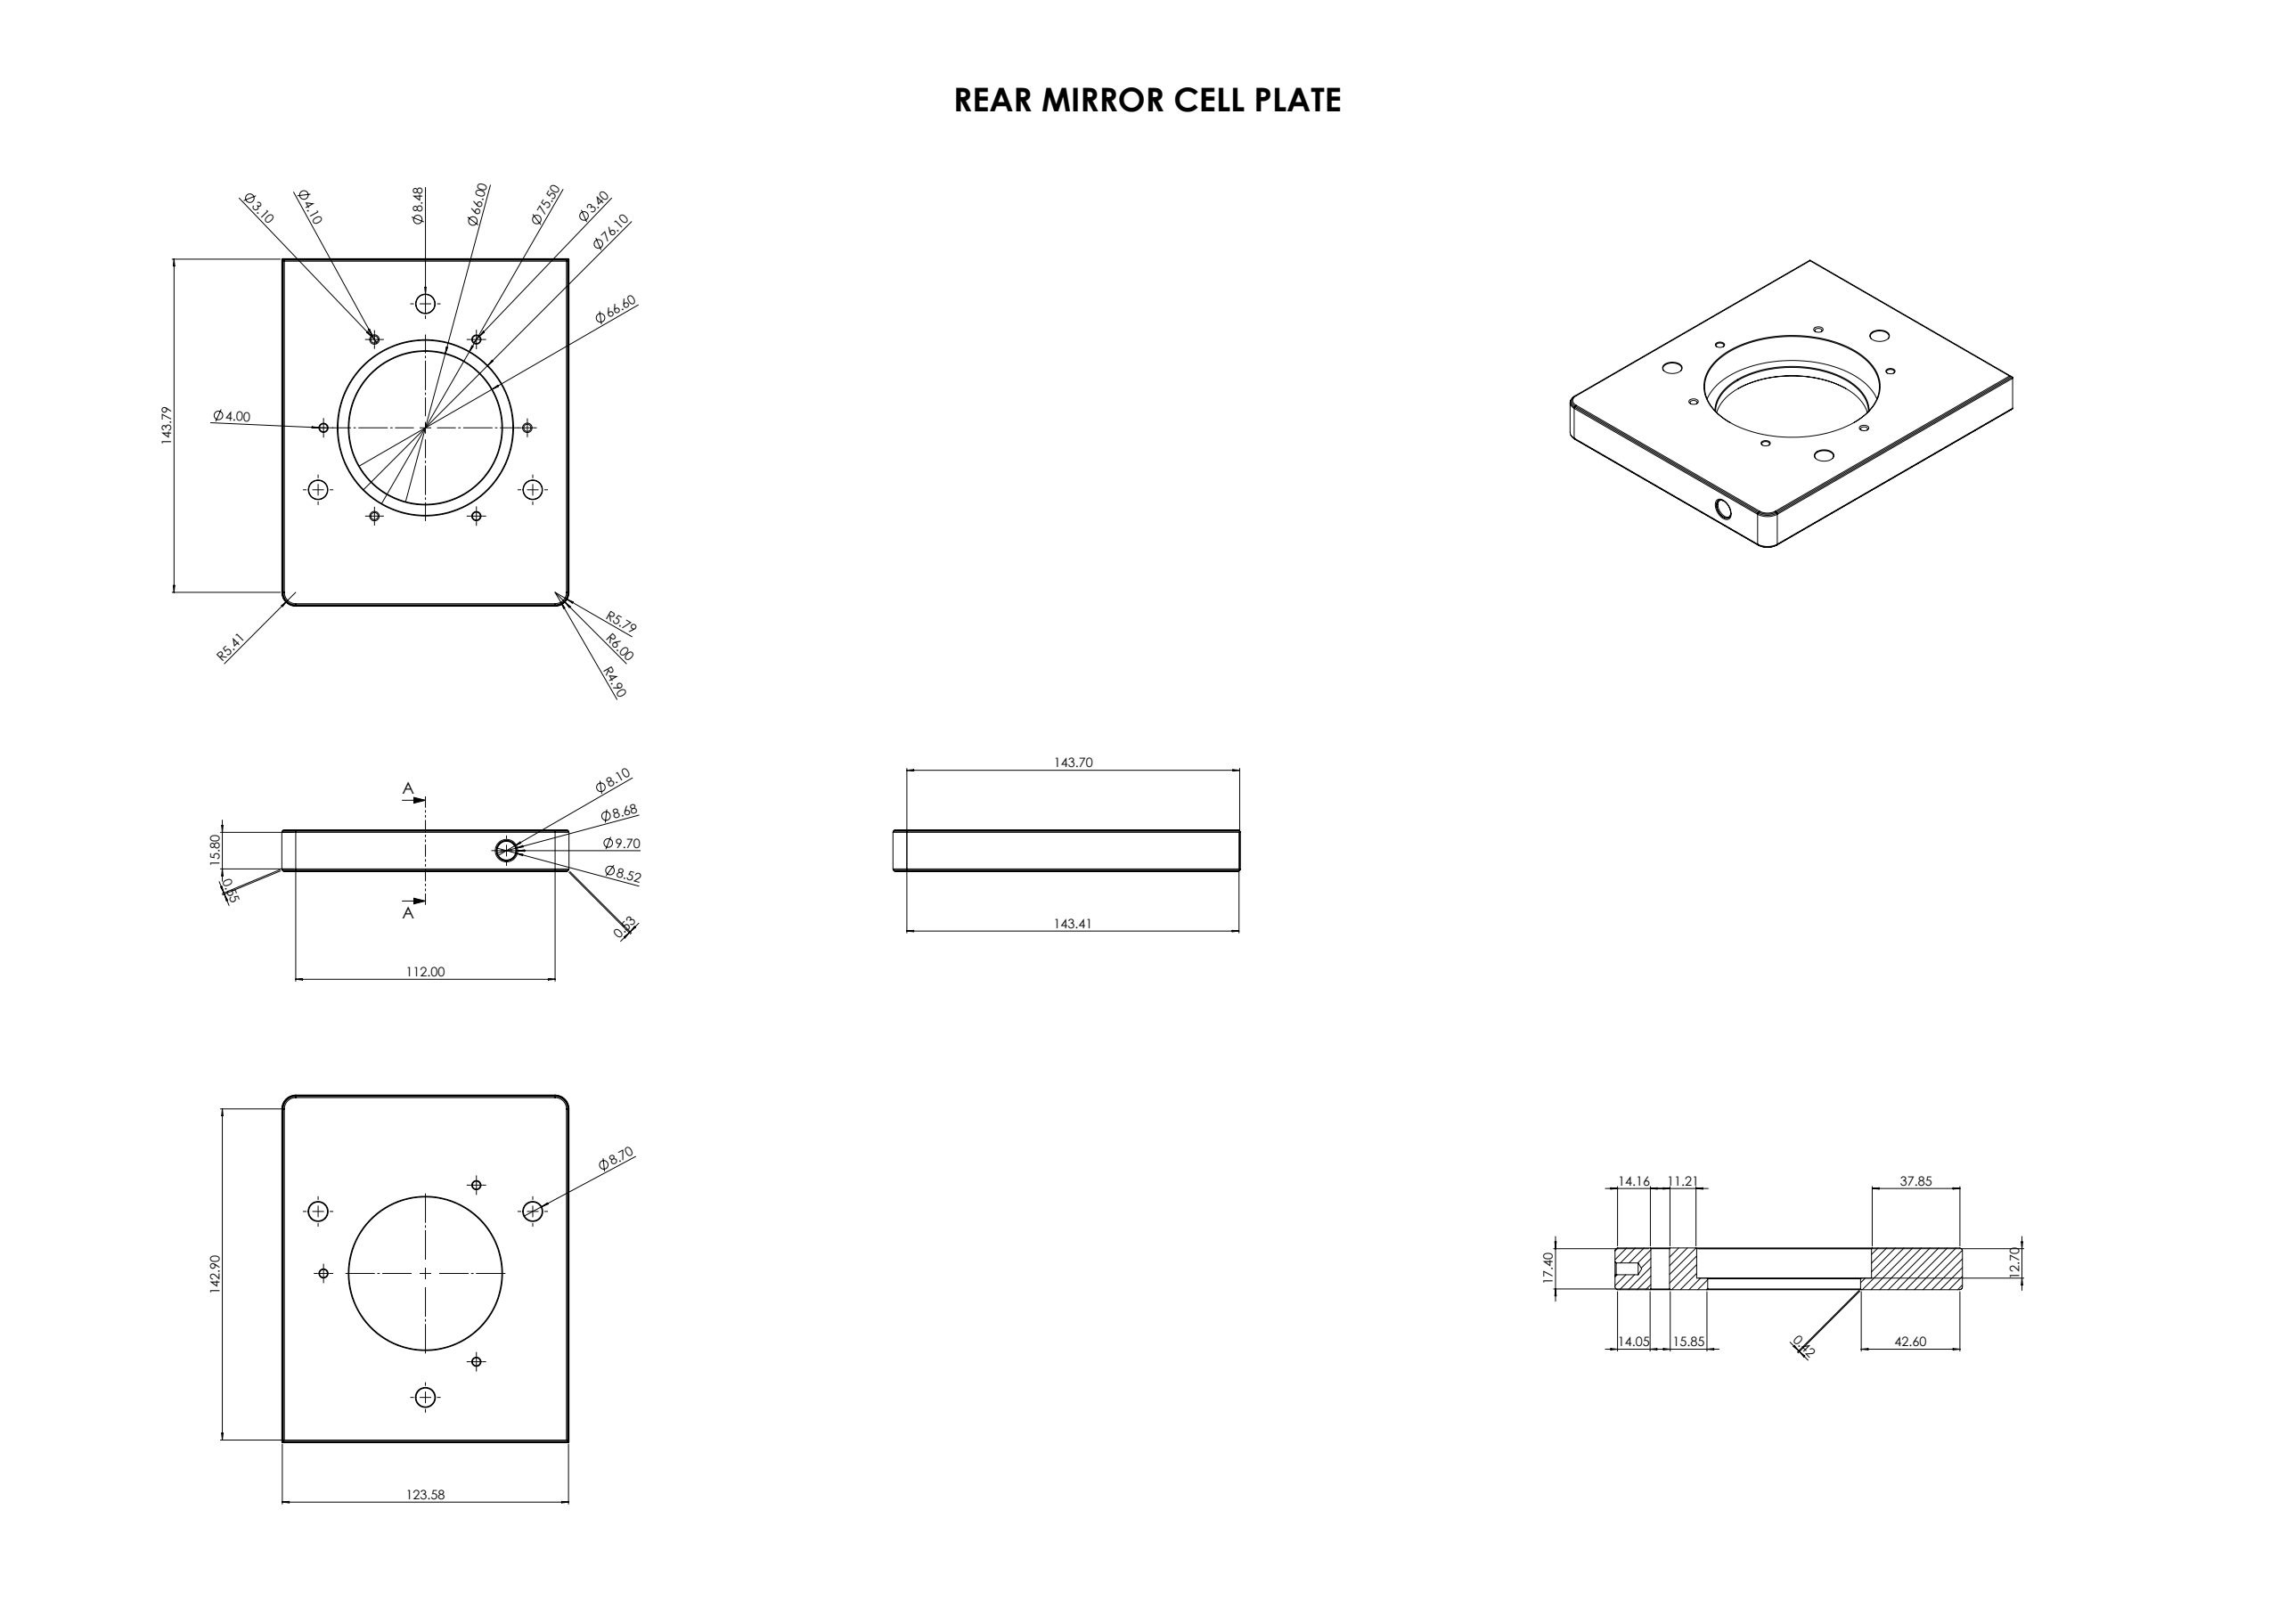
ISO-10303-21;
HEADER;
/* Generated by software containing ST-Developer
 * from STEP Tools, Inc. (www.steptools.com) 
 */

FILE_DESCRIPTION(
/* description */ (''),
/* implementation_level */ '2;1');

FILE_NAME(
/* name */ '02_Rear_Mirror_Cell_Plate.step',
/* time_stamp */ '2026-10-19T22:59:19-07:00',
/* author */ (''),
/* organization */ (''),
/* preprocessor_version */ 'ST-DEVELOPER v20.2',
/* originating_system */ 'Autodesk Translation Framework v15.15.0.0',
/* authorisation */ '');

FILE_SCHEMA (('AUTOMOTIVE_DESIGN { 1 0 10303 214 3 1 1 }'));
ENDSEC;

DATA;
#10=MECHANICAL_DESIGN_GEOMETRIC_PRESENTATION_REPRESENTATION('',(#912),#53650);
#880=SHAPE_REPRESENTATION_RELATIONSHIP('SRR','None',#53725,#896);
#896=ADVANCED_BREP_SHAPE_REPRESENTATION('',(#928),#53635);
#912=STYLED_ITEM('',(#53944),#928);
#928=MANIFOLD_SOLID_BREP('Rear Mirror Cell Plate',#23304);
#961=CYLINDRICAL_SURFACE('',#23742,0.6);
#962=CYLINDRICAL_SURFACE('',#23768,3.3);
#963=CYLINDRICAL_SURFACE('',#23773,3.775);
#964=CYLINDRICAL_SURFACE('',#23781,0.17);
#965=CYLINDRICAL_SURFACE('',#23787,0.17);
#966=CYLINDRICAL_SURFACE('',#23793,0.17);
#967=CYLINDRICAL_SURFACE('',#23798,0.405);
#968=CYLINDRICAL_SURFACE('',#23802,0.404999999999999);
#969=CYLINDRICAL_SURFACE('',#23806,0.405);
#970=CYLINDRICAL_SURFACE('',#23818,0.405);
#971=CYLINDRICAL_SURFACE('',#23823,0.255);
#972=CYLINDRICAL_SURFACE('',#23828,0.255);
#973=CYLINDRICAL_SURFACE('',#23833,0.255);
#974=CYLINDRICAL_SURFACE('',#23841,0.155);
#975=CYLINDRICAL_SURFACE('',#23846,0.155);
#976=CYLINDRICAL_SURFACE('',#23851,0.155);
#977=CYLINDRICAL_SURFACE('',#23855,0.6);
#1298=FACE_BOUND('',#3695,.T.);
#1299=FACE_BOUND('',#3696,.T.);
#1300=FACE_BOUND('',#3697,.T.);
#1301=FACE_BOUND('',#3698,.T.);
#1302=FACE_BOUND('',#3699,.T.);
#1303=FACE_BOUND('',#3700,.T.);
#1304=FACE_BOUND('',#3701,.T.);
#1305=FACE_BOUND('',#3704,.T.);
#1306=FACE_BOUND('',#3705,.T.);
#1307=FACE_BOUND('',#3706,.T.);
#1308=FACE_BOUND('',#3738,.T.);
#1309=FACE_BOUND('',#3739,.T.);
#1310=FACE_BOUND('',#3740,.T.);
#1311=FACE_BOUND('',#3741,.T.);
#1312=FACE_BOUND('',#3742,.T.);
#1313=FACE_BOUND('',#3743,.T.);
#1314=FACE_BOUND('',#3744,.T.);
#1315=FACE_BOUND('',#3745,.T.);
#1316=FACE_BOUND('',#3746,.T.);
#1317=FACE_BOUND('',#3747,.T.);
#1318=FACE_BOUND('',#3754,.T.);
#1319=FACE_BOUND('',#3773,.T.);
#1485=PLANE('',#23687);
#1486=PLANE('',#23688);
#1487=PLANE('',#23692);
#1488=PLANE('',#23696);
#1489=PLANE('',#23699);
#1490=PLANE('',#23700);
#1491=PLANE('',#23701);
#1492=PLANE('',#23709);
#1493=PLANE('',#23710);
#1494=PLANE('',#23714);
#1495=PLANE('',#23715);
#1496=PLANE('',#23716);
#1497=PLANE('',#23719);
#1498=PLANE('',#23723);
#1499=PLANE('',#23725);
#1500=PLANE('',#23726);
#1501=PLANE('',#23727);
#1502=PLANE('',#23728);
#1503=PLANE('',#23729);
#1504=PLANE('',#23730);
#1505=PLANE('',#23734);
#1506=PLANE('',#23740);
#1507=PLANE('',#23741);
#1508=PLANE('',#23743);
#1509=PLANE('',#23744);
#1510=PLANE('',#23745);
#1511=PLANE('',#23748);
#1512=PLANE('',#23752);
#1513=PLANE('',#23754);
#1514=PLANE('',#23755);
#1515=PLANE('',#23777);
#1516=PLANE('',#23814);
#1517=PLANE('',#23854);
#2336=FACE_OUTER_BOUND('',#3685,.T.);
#2337=FACE_OUTER_BOUND('',#3686,.T.);
#2338=FACE_OUTER_BOUND('',#3687,.T.);
#2339=FACE_OUTER_BOUND('',#3688,.T.);
#2340=FACE_OUTER_BOUND('',#3689,.T.);
#2341=FACE_OUTER_BOUND('',#3690,.T.);
#2342=FACE_OUTER_BOUND('',#3691,.T.);
#2343=FACE_OUTER_BOUND('',#3692,.T.);
#2344=FACE_OUTER_BOUND('',#3693,.T.);
#2345=FACE_OUTER_BOUND('',#3694,.T.);
#2346=FACE_OUTER_BOUND('',#3702,.T.);
#2347=FACE_OUTER_BOUND('',#3703,.T.);
#2348=FACE_OUTER_BOUND('',#3707,.T.);
#2349=FACE_OUTER_BOUND('',#3708,.T.);
#2350=FACE_OUTER_BOUND('',#3709,.T.);
#2351=FACE_OUTER_BOUND('',#3710,.T.);
#2352=FACE_OUTER_BOUND('',#3711,.T.);
#2353=FACE_OUTER_BOUND('',#3712,.T.);
#2354=FACE_OUTER_BOUND('',#3713,.T.);
#2355=FACE_OUTER_BOUND('',#3714,.T.);
#2356=FACE_OUTER_BOUND('',#3715,.T.);
#2357=FACE_OUTER_BOUND('',#3716,.T.);
#2358=FACE_OUTER_BOUND('',#3717,.T.);
#2359=FACE_OUTER_BOUND('',#3718,.T.);
#2360=FACE_OUTER_BOUND('',#3719,.T.);
#2361=FACE_OUTER_BOUND('',#3720,.T.);
#2362=FACE_OUTER_BOUND('',#3721,.T.);
#2363=FACE_OUTER_BOUND('',#3722,.T.);
#2364=FACE_OUTER_BOUND('',#3723,.T.);
#2365=FACE_OUTER_BOUND('',#3724,.T.);
#2366=FACE_OUTER_BOUND('',#3725,.T.);
#2367=FACE_OUTER_BOUND('',#3726,.T.);
#2368=FACE_OUTER_BOUND('',#3727,.T.);
#2369=FACE_OUTER_BOUND('',#3728,.T.);
#2370=FACE_OUTER_BOUND('',#3729,.T.);
#2371=FACE_OUTER_BOUND('',#3730,.T.);
#2372=FACE_OUTER_BOUND('',#3731,.T.);
#2373=FACE_OUTER_BOUND('',#3732,.T.);
#2374=FACE_OUTER_BOUND('',#3733,.T.);
#2375=FACE_OUTER_BOUND('',#3734,.T.);
#2376=FACE_OUTER_BOUND('',#3735,.T.);
#2377=FACE_OUTER_BOUND('',#3736,.T.);
#2378=FACE_OUTER_BOUND('',#3737,.T.);
#2379=FACE_OUTER_BOUND('',#3748,.T.);
#2380=FACE_OUTER_BOUND('',#3749,.T.);
#2381=FACE_OUTER_BOUND('',#3750,.T.);
#2382=FACE_OUTER_BOUND('',#3751,.T.);
#2383=FACE_OUTER_BOUND('',#3752,.T.);
#2384=FACE_OUTER_BOUND('',#3753,.T.);
#2385=FACE_OUTER_BOUND('',#3755,.T.);
#2386=FACE_OUTER_BOUND('',#3756,.T.);
#2387=FACE_OUTER_BOUND('',#3757,.T.);
#2388=FACE_OUTER_BOUND('',#3758,.T.);
#2389=FACE_OUTER_BOUND('',#3759,.T.);
#2390=FACE_OUTER_BOUND('',#3760,.T.);
#2391=FACE_OUTER_BOUND('',#3761,.T.);
#2392=FACE_OUTER_BOUND('',#3762,.T.);
#2393=FACE_OUTER_BOUND('',#3763,.T.);
#2394=FACE_OUTER_BOUND('',#3764,.T.);
#2395=FACE_OUTER_BOUND('',#3765,.T.);
#2396=FACE_OUTER_BOUND('',#3766,.T.);
#2397=FACE_OUTER_BOUND('',#3767,.T.);
#2398=FACE_OUTER_BOUND('',#3768,.T.);
#2399=FACE_OUTER_BOUND('',#3769,.T.);
#2400=FACE_OUTER_BOUND('',#3770,.T.);
#2401=FACE_OUTER_BOUND('',#3771,.T.);
#2402=FACE_OUTER_BOUND('',#3772,.T.);
#2403=FACE_OUTER_BOUND('',#3774,.T.);
#2404=FACE_OUTER_BOUND('',#3775,.T.);
#2405=FACE_OUTER_BOUND('',#3776,.T.);
#2406=FACE_OUTER_BOUND('',#3777,.T.);
#2407=FACE_OUTER_BOUND('',#3778,.T.);
#2408=FACE_OUTER_BOUND('',#3779,.T.);
#2409=FACE_OUTER_BOUND('',#3780,.T.);
#2410=FACE_OUTER_BOUND('',#3781,.T.);
#2411=FACE_OUTER_BOUND('',#3782,.T.);
#2412=FACE_OUTER_BOUND('',#3783,.T.);
#2413=FACE_OUTER_BOUND('',#3784,.T.);
#2414=FACE_OUTER_BOUND('',#3785,.T.);
#2415=FACE_OUTER_BOUND('',#3786,.T.);
#2416=FACE_OUTER_BOUND('',#3787,.T.);
#2417=FACE_OUTER_BOUND('',#3788,.T.);
#2418=FACE_OUTER_BOUND('',#3789,.T.);
#2419=FACE_OUTER_BOUND('',#3790,.T.);
#2420=FACE_OUTER_BOUND('',#3791,.T.);
#2421=FACE_OUTER_BOUND('',#3792,.T.);
#2422=FACE_OUTER_BOUND('',#3793,.T.);
#2423=FACE_OUTER_BOUND('',#3794,.T.);
#2424=FACE_OUTER_BOUND('',#3795,.T.);
#2425=FACE_OUTER_BOUND('',#3796,.T.);
#2426=FACE_OUTER_BOUND('',#3797,.T.);
#2427=FACE_OUTER_BOUND('',#3798,.T.);
#2428=FACE_OUTER_BOUND('',#3799,.T.);
#3685=EDGE_LOOP('',(#15489,#15490,#15491,#15492));
#3686=EDGE_LOOP('',(#15493,#15494,#15495,#15496));
#3687=EDGE_LOOP('',(#15497,#15498,#15499,#15500));
#3688=EDGE_LOOP('',(#15501,#15502,#15503,#15504));
#3689=EDGE_LOOP('',(#15505,#15506,#15507,#15508));
#3690=EDGE_LOOP('',(#15509,#15510,#15511,#15512));
#3691=EDGE_LOOP('',(#15513,#15514,#15515,#15516));
#3692=EDGE_LOOP('',(#15517,#15518,#15519,#15520));
#3693=EDGE_LOOP('',(#15521,#15522,#15523,#15524));
#3694=EDGE_LOOP('',(#15525,#15526,#15527,#15528,#15529,#15530));
#3695=EDGE_LOOP('',(#15531));
#3696=EDGE_LOOP('',(#15532));
#3697=EDGE_LOOP('',(#15533));
#3698=EDGE_LOOP('',(#15534));
#3699=EDGE_LOOP('',(#15535));
#3700=EDGE_LOOP('',(#15536));
#3701=EDGE_LOOP('',(#15537));
#3702=EDGE_LOOP('',(#15538,#15539,#15540,#15541,#15542,#15543));
#3703=EDGE_LOOP('',(#15544,#15545,#15546,#15547));
#3704=EDGE_LOOP('',(#15548));
#3705=EDGE_LOOP('',(#15549));
#3706=EDGE_LOOP('',(#15550));
#3707=EDGE_LOOP('',(#15551,#15552,#15553,#15554,#15555,#15556));
#3708=EDGE_LOOP('',(#15557,#15558,#15559,#15560,#15561));
#3709=EDGE_LOOP('',(#15562,#15563,#15564,#15565,#15566));
#3710=EDGE_LOOP('',(#15567,#15568,#15569,#15570));
#3711=EDGE_LOOP('',(#15571,#15572,#15573,#15574));
#3712=EDGE_LOOP('',(#15575,#15576,#15577,#15578));
#3713=EDGE_LOOP('',(#15579,#15580,#15581,#15582));
#3714=EDGE_LOOP('',(#15583,#15584,#15585,#15586));
#3715=EDGE_LOOP('',(#15587,#15588,#15589,#15590));
#3716=EDGE_LOOP('',(#15591,#15592,#15593,#15594,#15595,#15596));
#3717=EDGE_LOOP('',(#15597,#15598,#15599,#15600,#15601,#15602));
#3718=EDGE_LOOP('',(#15603,#15604,#15605,#15606));
#3719=EDGE_LOOP('',(#15607,#15608,#15609,#15610,#15611));
#3720=EDGE_LOOP('',(#15612,#15613,#15614,#15615,#15616));
#3721=EDGE_LOOP('',(#15617,#15618,#15619,#15620));
#3722=EDGE_LOOP('',(#15621,#15622,#15623,#15624));
#3723=EDGE_LOOP('',(#15625,#15626,#15627,#15628));
#3724=EDGE_LOOP('',(#15629,#15630,#15631,#15632));
#3725=EDGE_LOOP('',(#15633,#15634,#15635,#15636));
#3726=EDGE_LOOP('',(#15637,#15638,#15639,#15640));
#3727=EDGE_LOOP('',(#15641,#15642,#15643,#15644));
#3728=EDGE_LOOP('',(#15645,#15646,#15647,#15648));
#3729=EDGE_LOOP('',(#15649,#15650,#15651,#15652));
#3730=EDGE_LOOP('',(#15653,#15654,#15655,#15656));
#3731=EDGE_LOOP('',(#15657,#15658,#15659,#15660));
#3732=EDGE_LOOP('',(#15661,#15662,#15663,#15664));
#3733=EDGE_LOOP('',(#15665,#15666,#15667,#15668));
#3734=EDGE_LOOP('',(#15669,#15670,#15671,#15672));
#3735=EDGE_LOOP('',(#15673,#15674,#15675,#15676));
#3736=EDGE_LOOP('',(#15677,#15678,#15679,#15680));
#3737=EDGE_LOOP('',(#15681,#15682,#15683,#15684,#15685,#15686));
#3738=EDGE_LOOP('',(#15687));
#3739=EDGE_LOOP('',(#15688));
#3740=EDGE_LOOP('',(#15689));
#3741=EDGE_LOOP('',(#15690));
#3742=EDGE_LOOP('',(#15691));
#3743=EDGE_LOOP('',(#15692));
#3744=EDGE_LOOP('',(#15693));
#3745=EDGE_LOOP('',(#15694));
#3746=EDGE_LOOP('',(#15695));
#3747=EDGE_LOOP('',(#15696));
#3748=EDGE_LOOP('',(#15697,#15698,#15699,#15700));
#3749=EDGE_LOOP('',(#15701,#15702,#15703,#15704));
#3750=EDGE_LOOP('',(#15705,#15706,#15707,#15708,#15709));
#3751=EDGE_LOOP('',(#15710,#15711,#15712,#15713,#15714));
#3752=EDGE_LOOP('',(#15715,#15716,#15717,#15718));
#3753=EDGE_LOOP('',(#15719));
#3754=EDGE_LOOP('',(#15720));
#3755=EDGE_LOOP('',(#15721,#15722,#15723,#15724,#15725));
#3756=EDGE_LOOP('',(#15726,#15727,#15728,#15729,#15730));
#3757=EDGE_LOOP('',(#15731,#15732,#15733,#15734));
#3758=EDGE_LOOP('',(#15735,#15736,#15737,#15738,#15739));
#3759=EDGE_LOOP('',(#15740,#15741,#15742,#15743,#15744));
#3760=EDGE_LOOP('',(#15745,#15746,#15747,#15748));
#3761=EDGE_LOOP('',(#15749,#15750,#15751,#15752,#15753));
#3762=EDGE_LOOP('',(#15754,#15755,#15756,#15757,#15758));
#3763=EDGE_LOOP('',(#15759,#15760,#15761,#15762));
#3764=EDGE_LOOP('',(#15763,#15764,#15765,#15766));
#3765=EDGE_LOOP('',(#15767,#15768,#15769,#15770));
#3766=EDGE_LOOP('',(#15771,#15772,#15773,#15774));
#3767=EDGE_LOOP('',(#15775,#15776,#15777,#15778));
#3768=EDGE_LOOP('',(#15779,#15780,#15781,#15782));
#3769=EDGE_LOOP('',(#15783,#15784,#15785,#15786));
#3770=EDGE_LOOP('',(#15787,#15788,#15789,#15790));
#3771=EDGE_LOOP('',(#15791,#15792,#15793,#15794,#15795));
#3772=EDGE_LOOP('',(#15796,#15797,#15798,#15799));
#3773=EDGE_LOOP('',(#15800));
#3774=EDGE_LOOP('',(#15801,#15802,#15803,#15804,#15805,#15806));
#3775=EDGE_LOOP('',(#15807,#15808,#15809,#15810,#15811));
#3776=EDGE_LOOP('',(#15812,#15813,#15814));
#3777=EDGE_LOOP('',(#15815,#15816,#15817));
#3778=EDGE_LOOP('',(#15818,#15819,#15820,#15821));
#3779=EDGE_LOOP('',(#15822,#15823,#15824,#15825));
#3780=EDGE_LOOP('',(#15826,#15827,#15828));
#3781=EDGE_LOOP('',(#15829,#15830,#15831,#15832));
#3782=EDGE_LOOP('',(#15833,#15834,#15835,#15836));
#3783=EDGE_LOOP('',(#15837,#15838,#15839));
#3784=EDGE_LOOP('',(#15840,#15841,#15842,#15843));
#3785=EDGE_LOOP('',(#15844,#15845,#15846,#15847));
#3786=EDGE_LOOP('',(#15848,#15849,#15850,#15851));
#3787=EDGE_LOOP('',(#15852,#15853,#15854,#15855));
#3788=EDGE_LOOP('',(#15856,#15857,#15858,#15859));
#3789=EDGE_LOOP('',(#15860,#15861,#15862));
#3790=EDGE_LOOP('',(#15863,#15864,#15865,#15866));
#3791=EDGE_LOOP('',(#15867,#15868,#15869,#15870));
#3792=EDGE_LOOP('',(#15871,#15872,#15873));
#3793=EDGE_LOOP('',(#15874,#15875,#15876,#15877));
#3794=EDGE_LOOP('',(#15878,#15879,#15880,#15881));
#3795=EDGE_LOOP('',(#15882,#15883,#15884));
#3796=EDGE_LOOP('',(#15885,#15886,#15887,#15888));
#3797=EDGE_LOOP('',(#15889,#15890,#15891,#15892));
#3798=EDGE_LOOP('',(#15893,#15894,#15895,#15896));
#3799=EDGE_LOOP('',(#15897,#15898,#15899,#15900));
#5151=CIRCLE('',#23690,0.541213203435597);
#5152=CIRCLE('',#23691,0.49);
#5153=CIRCLE('',#23694,0.541213203435596);
#5154=CIRCLE('',#23695,0.489999999999998);
#5155=CIRCLE('',#23698,0.578786796564402);
#5156=CIRCLE('',#23702,3.33);
#5157=CIRCLE('',#23703,0.2);
#5158=CIRCLE('',#23704,0.435);
#5159=CIRCLE('',#23705,0.435);
#5160=CIRCLE('',#23706,0.435);
#5161=CIRCLE('',#23707,0.2);
#5162=CIRCLE('',#23708,0.2);
#5163=CIRCLE('',#23711,0.305);
#5164=CIRCLE('',#23712,0.305);
#5165=CIRCLE('',#23713,0.305);
#5166=CIRCLE('',#23718,0.6);
#5167=CIRCLE('',#23721,0.578786796564403);
#5168=CIRCLE('',#23722,0.6);
#5169=CIRCLE('',#23732,0.578786796564403);
#5170=CIRCLE('',#23733,0.6);
#5171=CIRCLE('',#23736,0.578786796564403);
#5172=CIRCLE('',#23737,0.6);
#5173=CIRCLE('',#23739,0.541213203435596);
#5174=CIRCLE('',#23747,0.489999999999998);
#5175=CIRCLE('',#23750,0.541213203435597);
#5176=CIRCLE('',#23751,0.49);
#5177=CIRCLE('',#23756,3.805);
#5178=CIRCLE('',#23757,0.2);
#5179=CIRCLE('',#23758,0.42375);
#5180=CIRCLE('',#23759,0.423750000000001);
#5181=CIRCLE('',#23760,0.205);
#5182=CIRCLE('',#23761,0.205000000000001);
#5183=CIRCLE('',#23762,0.205);
#5184=CIRCLE('',#23763,0.423749999999999);
#5185=CIRCLE('',#23764,0.2);
#5186=CIRCLE('',#23765,0.2);
#5187=CIRCLE('',#23767,3.3);
#5188=CIRCLE('',#23769,3.3);
#5189=CIRCLE('',#23771,3.775);
#5190=CIRCLE('',#23772,3.775);
#5191=CIRCLE('',#23774,3.775);
#5192=CIRCLE('',#23776,3.33);
#5193=CIRCLE('',#23779,0.17);
#5194=CIRCLE('',#23780,0.17);
#5195=CIRCLE('',#23782,0.17);
#5196=CIRCLE('',#23785,0.17);
#5197=CIRCLE('',#23786,0.17);
#5198=CIRCLE('',#23788,0.17);
#5199=CIRCLE('',#23791,0.17);
#5200=CIRCLE('',#23792,0.17);
#5201=CIRCLE('',#23794,0.17);
#5202=CIRCLE('',#23797,0.405);
#5203=CIRCLE('',#23799,0.405);
#5204=CIRCLE('',#23801,0.404999999999999);
#5205=CIRCLE('',#23803,0.404999999999999);
#5206=CIRCLE('',#23805,0.405);
#5207=CIRCLE('',#23807,0.405);
#5208=CIRCLE('',#23809,0.485000000000001);
#5209=CIRCLE('',#23810,0.433786796564405);
#5210=CIRCLE('',#23812,0.426213203435597);
#5211=CIRCLE('',#23813,0.426213203435597);
#5212=CIRCLE('',#23816,0.405);
#5213=CIRCLE('',#23817,0.405);
#5214=CIRCLE('',#23819,0.405);
#5215=CIRCLE('',#23822,0.255);
#5216=CIRCLE('',#23824,0.255);
#5217=CIRCLE('',#23827,0.255);
#5218=CIRCLE('',#23829,0.255);
#5219=CIRCLE('',#23832,0.255);
#5220=CIRCLE('',#23834,0.255);
#5221=CIRCLE('',#23840,0.155);
#5222=CIRCLE('',#23842,0.155);
#5223=CIRCLE('',#23845,0.155);
#5224=CIRCLE('',#23847,0.155);
#5225=CIRCLE('',#23850,0.155);
#5226=CIRCLE('',#23852,0.155);
#5975=LINE('',#32252,#7820);
#5976=LINE('',#32254,#7821);
#5977=LINE('',#32256,#7822);
#5978=LINE('',#32257,#7823);
#5979=LINE('',#32260,#7824);
#5980=LINE('',#32262,#7825);
#5981=LINE('',#32263,#7826);
#5982=LINE('',#32267,#7827);
#5983=LINE('',#32273,#7828);
#5984=LINE('',#32274,#7829);
#5985=LINE('',#32275,#7830);
#5986=LINE('',#32279,#7831);
#5987=LINE('',#32283,#7832);
#5988=LINE('',#32284,#7833);
#5989=LINE('',#32287,#7834);
#5990=LINE('',#32290,#7835);
#5991=LINE('',#32293,#7836);
#5992=LINE('',#32294,#7837);
#5993=LINE('',#32297,#7838);
#5994=LINE('',#32298,#7839);
#5995=LINE('',#32316,#7840);
#5996=LINE('',#32318,#7841);
#5997=LINE('',#32320,#7842);
#5998=LINE('',#32322,#7843);
#5999=LINE('',#32323,#7844);
#6000=LINE('',#32326,#7845);
#6001=LINE('',#32328,#7846);
#6002=LINE('',#32329,#7847);
#6003=LINE('',#32338,#7848);
#6004=LINE('',#32340,#7849);
#6005=LINE('',#32342,#7850);
#6006=LINE('',#32343,#7851);
#6007=LINE('',#32346,#7852);
#6008=LINE('',#32348,#7853);
#6009=LINE('',#32349,#7854);
#6010=LINE('',#32352,#7855);
#6011=LINE('',#32354,#7856);
#6012=LINE('',#32355,#7857);
#6013=LINE('',#32358,#7858);
#6014=LINE('',#32363,#7859);
#6015=LINE('',#32364,#7860);
#6016=LINE('',#32365,#7861);
#6017=LINE('',#32370,#7862);
#6018=LINE('',#32372,#7863);
#6019=LINE('',#32376,#7864);
#6020=LINE('',#32378,#7865);
#6021=LINE('',#32380,#7866);
#6022=LINE('',#32381,#7867);
#6023=LINE('',#32384,#7868);
#6024=LINE('',#32385,#7869);
#6025=LINE('',#32388,#7870);
#6026=LINE('',#32389,#7871);
#6027=LINE('',#32392,#7872);
#6028=LINE('',#32393,#7873);
#6029=LINE('',#32396,#7874);
#6030=LINE('',#32398,#7875);
#6031=LINE('',#32399,#7876);
#6032=LINE('',#32403,#7877);
#6033=LINE('',#32409,#7878);
#6034=LINE('',#32410,#7879);
#6035=LINE('',#32411,#7880);
#6036=LINE('',#32417,#7881);
#6037=LINE('',#32420,#7882);
#6038=LINE('',#32423,#7883);
#6039=LINE('',#32424,#7884);
#6040=LINE('',#32427,#7885);
#6041=LINE('',#32428,#7886);
#6042=LINE('',#32430,#7887);
#6043=LINE('',#32431,#7888);
#6044=LINE('',#32436,#7889);
#6045=LINE('',#32437,#7890);
#6046=LINE('',#32438,#7891);
#6047=LINE('',#32441,#7892);
#6048=LINE('',#32442,#7893);
#6049=LINE('',#32445,#7894);
#6050=LINE('',#32450,#7895);
#6051=LINE('',#32451,#7896);
#6052=LINE('',#32452,#7897);
#6053=LINE('',#32456,#7898);
#6054=LINE('',#32460,#7899);
#6055=LINE('',#32461,#7900);
#6056=LINE('',#32463,#7901);
#6057=LINE('',#32464,#7902);
#6058=LINE('',#32489,#7903);
#6059=LINE('',#32493,#7904);
#6060=LINE('',#32497,#7905);
#6061=LINE('',#32504,#7906);
#6062=LINE('',#32507,#7907);
#6063=LINE('',#32512,#7908);
#6064=LINE('',#32519,#7909);
#6065=LINE('',#32521,#7910);
#6066=LINE('',#32524,#7911);
#6067=LINE('',#32531,#7912);
#6068=LINE('',#32533,#7913);
#6069=LINE('',#32536,#7914);
#6070=LINE('',#32543,#7915);
#6071=LINE('',#32545,#7916);
#6072=LINE('',#32548,#7917);
#6073=LINE('',#32552,#7918);
#6074=LINE('',#32556,#7919);
#6075=LINE('',#32560,#7920);
#6076=LINE('',#32564,#7921);
#6077=LINE('',#32568,#7922);
#6078=LINE('',#32574,#7923);
#6079=LINE('',#32581,#7924);
#6080=LINE('',#32583,#7925);
#6081=LINE('',#32589,#7926);
#6082=LINE('',#32593,#7927);
#6083=LINE('',#32596,#7928);
#6084=LINE('',#32600,#7929);
#6085=LINE('',#32604,#7930);
#6086=LINE('',#32607,#7931);
#6087=LINE('',#32611,#7932);
#6088=LINE('',#32615,#7933);
#6089=LINE('',#32618,#7934);
#6090=LINE('',#32622,#7935);
#6091=LINE('',#32626,#7936);
#6092=LINE('',#32629,#7937);
#6093=LINE('',#32631,#7938);
#6094=LINE('',#32633,#7939);
#6095=LINE('',#32635,#7940);
#6096=LINE('',#32639,#7941);
#6097=LINE('',#32643,#7942);
#6098=LINE('',#32646,#7943);
#6099=LINE('',#32650,#7944);
#6100=LINE('',#32654,#7945);
#6101=LINE('',#32657,#7946);
#6102=LINE('',#32661,#7947);
#6103=LINE('',#32665,#7948);
#6104=LINE('',#32668,#7949);
#7820=VECTOR('',#26161,1.);
#7821=VECTOR('',#26162,1.);
#7822=VECTOR('',#26163,1.);
#7823=VECTOR('',#26164,1.);
#7824=VECTOR('',#26167,1.);
#7825=VECTOR('',#26168,1.);
#7826=VECTOR('',#26169,1.);
#7827=VECTOR('',#26172,1.);
#7828=VECTOR('',#26179,1.);
#7829=VECTOR('',#26180,1.);
#7830=VECTOR('',#26181,1.);
#7831=VECTOR('',#26184,1.);
#7832=VECTOR('',#26191,1.);
#7833=VECTOR('',#26192,1.);
#7834=VECTOR('',#26195,1.);
#7835=VECTOR('',#26198,1.);
#7836=VECTOR('',#26201,1.);
#7837=VECTOR('',#26202,1.);
#7838=VECTOR('',#26205,1.);
#7839=VECTOR('',#26206,1.);
#7840=VECTOR('',#26225,1.);
#7841=VECTOR('',#26226,1.);
#7842=VECTOR('',#26227,1.);
#7843=VECTOR('',#26228,1.);
#7844=VECTOR('',#26229,1.);
#7845=VECTOR('',#26232,1.);
#7846=VECTOR('',#26233,1.);
#7847=VECTOR('',#26234,1.);
#7848=VECTOR('',#26243,1.);
#7849=VECTOR('',#26244,1.);
#7850=VECTOR('',#26245,1.);
#7851=VECTOR('',#26246,1.);
#7852=VECTOR('',#26249,1.);
#7853=VECTOR('',#26250,1.);
#7854=VECTOR('',#26251,1.);
#7855=VECTOR('',#26254,1.);
#7856=VECTOR('',#26255,1.);
#7857=VECTOR('',#26256,1.);
#7858=VECTOR('',#26259,1.);
#7859=VECTOR('',#26264,1.);
#7860=VECTOR('',#26265,1.);
#7861=VECTOR('',#26266,1.);
#7862=VECTOR('',#26275,1.);
#7863=VECTOR('',#26278,1.);
#7864=VECTOR('',#26283,1.);
#7865=VECTOR('',#26284,1.);
#7866=VECTOR('',#26285,1.);
#7867=VECTOR('',#26286,1.);
#7868=VECTOR('',#26289,1.);
#7869=VECTOR('',#26290,1.);
#7870=VECTOR('',#26293,1.);
#7871=VECTOR('',#26294,1.);
#7872=VECTOR('',#26297,1.);
#7873=VECTOR('',#26298,1.);
#7874=VECTOR('',#26301,1.);
#7875=VECTOR('',#26302,1.);
#7876=VECTOR('',#26303,1.);
#7877=VECTOR('',#26306,1.);
#7878=VECTOR('',#26313,1.);
#7879=VECTOR('',#26314,1.);
#7880=VECTOR('',#26315,1.);
#7881=VECTOR('',#26324,1.);
#7882=VECTOR('',#26327,1.);
#7883=VECTOR('',#26330,1.);
#7884=VECTOR('',#26331,1.);
#7885=VECTOR('',#26334,1.);
#7886=VECTOR('',#26335,1.);
#7887=VECTOR('',#26338,1.);
#7888=VECTOR('',#26339,1.);
#7889=VECTOR('',#26344,1.);
#7890=VECTOR('',#26345,1.);
#7891=VECTOR('',#26346,1.);
#7892=VECTOR('',#26349,1.);
#7893=VECTOR('',#26350,1.);
#7894=VECTOR('',#26353,1.);
#7895=VECTOR('',#26358,1.);
#7896=VECTOR('',#26359,1.);
#7897=VECTOR('',#26360,1.);
#7898=VECTOR('',#26363,1.);
#7899=VECTOR('',#26370,1.);
#7900=VECTOR('',#26371,1.);
#7901=VECTOR('',#26374,1.);
#7902=VECTOR('',#26375,1.);
#7903=VECTOR('',#26402,3.315);
#7904=VECTOR('',#26407,3.3);
#7905=VECTOR('',#26412,3.79);
#7906=VECTOR('',#26421,3.775);
#7907=VECTOR('',#26424,3.315);
#7908=VECTOR('',#26431,0.185);
#7909=VECTOR('',#26440,0.17);
#7910=VECTOR('',#26443,0.185);
#7911=VECTOR('',#26446,0.185);
#7912=VECTOR('',#26455,0.17);
#7913=VECTOR('',#26458,0.185);
#7914=VECTOR('',#26461,0.185);
#7915=VECTOR('',#26470,0.17);
#7916=VECTOR('',#26473,0.185);
#7917=VECTOR('',#26476,0.42);
#7918=VECTOR('',#26481,0.405);
#7919=VECTOR('',#26486,0.42);
#7920=VECTOR('',#26491,0.404999999999999);
#7921=VECTOR('',#26496,0.42);
#7922=VECTOR('',#26501,0.405);
#7923=VECTOR('',#26508,0.459393398282203);
#7924=VECTOR('',#26517,0.455);
#7925=VECTOR('',#26520,1.);
#7926=VECTOR('',#26527,0.415606601717798);
#7927=VECTOR('',#26532,0.405);
#7928=VECTOR('',#26535,0.2025);
#7929=VECTOR('',#26538,0.1275);
#7930=VECTOR('',#26543,0.255);
#7931=VECTOR('',#26548,0.305);
#7932=VECTOR('',#26551,0.1275);
#7933=VECTOR('',#26556,0.255);
#7934=VECTOR('',#26561,0.305);
#7935=VECTOR('',#26564,0.1275);
#7936=VECTOR('',#26569,0.255);
#7937=VECTOR('',#26574,0.305);
#7938=VECTOR('',#26577,0.43);
#7939=VECTOR('',#26580,0.429999999999999);
#7940=VECTOR('',#26583,0.430000000000001);
#7941=VECTOR('',#26586,0.0775000000000001);
#7942=VECTOR('',#26591,0.155);
#7943=VECTOR('',#26596,0.205);
#7944=VECTOR('',#26599,0.0775000000000001);
#7945=VECTOR('',#26604,0.155);
#7946=VECTOR('',#26609,0.205000000000001);
#7947=VECTOR('',#26612,0.0775000000000006);
#7948=VECTOR('',#26617,0.155);
#7949=VECTOR('',#26622,0.205);
#9662=VERTEX_POINT('',#32250);
#9663=VERTEX_POINT('',#32251);
#9664=VERTEX_POINT('',#32253);
#9665=VERTEX_POINT('',#32255);
#9666=VERTEX_POINT('',#32259);
#9667=VERTEX_POINT('',#32261);
#9668=VERTEX_POINT('',#32265);
#9669=VERTEX_POINT('',#32266);
#9670=VERTEX_POINT('',#32271);
#9671=VERTEX_POINT('',#32272);
#9672=VERTEX_POINT('',#32277);
#9673=VERTEX_POINT('',#32278);
#9674=VERTEX_POINT('',#32286);
#9675=VERTEX_POINT('',#32288);
#9676=VERTEX_POINT('',#32292);
#9677=VERTEX_POINT('',#32296);
#9678=VERTEX_POINT('',#32300);
#9679=VERTEX_POINT('',#32302);
#9680=VERTEX_POINT('',#32304);
#9681=VERTEX_POINT('',#32306);
#9682=VERTEX_POINT('',#32308);
#9683=VERTEX_POINT('',#32310);
#9684=VERTEX_POINT('',#32312);
#9685=VERTEX_POINT('',#32315);
#9686=VERTEX_POINT('',#32317);
#9687=VERTEX_POINT('',#32319);
#9688=VERTEX_POINT('',#32321);
#9689=VERTEX_POINT('',#32325);
#9690=VERTEX_POINT('',#32327);
#9691=VERTEX_POINT('',#32330);
#9692=VERTEX_POINT('',#32332);
#9693=VERTEX_POINT('',#32334);
#9694=VERTEX_POINT('',#32337);
#9695=VERTEX_POINT('',#32339);
#9696=VERTEX_POINT('',#32341);
#9697=VERTEX_POINT('',#32345);
#9698=VERTEX_POINT('',#32347);
#9699=VERTEX_POINT('',#32351);
#9700=VERTEX_POINT('',#32353);
#9701=VERTEX_POINT('',#32357);
#9702=VERTEX_POINT('',#32361);
#9703=VERTEX_POINT('',#32362);
#9704=VERTEX_POINT('',#32375);
#9705=VERTEX_POINT('',#32377);
#9706=VERTEX_POINT('',#32379);
#9707=VERTEX_POINT('',#32383);
#9708=VERTEX_POINT('',#32387);
#9709=VERTEX_POINT('',#32391);
#9710=VERTEX_POINT('',#32395);
#9711=VERTEX_POINT('',#32397);
#9712=VERTEX_POINT('',#32401);
#9713=VERTEX_POINT('',#32402);
#9714=VERTEX_POINT('',#32407);
#9715=VERTEX_POINT('',#32408);
#9716=VERTEX_POINT('',#32416);
#9717=VERTEX_POINT('',#32418);
#9718=VERTEX_POINT('',#32422);
#9719=VERTEX_POINT('',#32426);
#9720=VERTEX_POINT('',#32434);
#9721=VERTEX_POINT('',#32435);
#9722=VERTEX_POINT('',#32440);
#9723=VERTEX_POINT('',#32444);
#9724=VERTEX_POINT('',#32448);
#9725=VERTEX_POINT('',#32449);
#9726=VERTEX_POINT('',#32454);
#9727=VERTEX_POINT('',#32455);
#9728=VERTEX_POINT('',#32467);
#9729=VERTEX_POINT('',#32469);
#9730=VERTEX_POINT('',#32471);
#9731=VERTEX_POINT('',#32473);
#9732=VERTEX_POINT('',#32475);
#9733=VERTEX_POINT('',#32477);
#9734=VERTEX_POINT('',#32479);
#9735=VERTEX_POINT('',#32481);
#9736=VERTEX_POINT('',#32483);
#9737=VERTEX_POINT('',#32485);
#9738=VERTEX_POINT('',#32488);
#9739=VERTEX_POINT('',#32492);
#9740=VERTEX_POINT('',#32496);
#9741=VERTEX_POINT('',#32498);
#9742=VERTEX_POINT('',#32502);
#9743=VERTEX_POINT('',#32506);
#9744=VERTEX_POINT('',#32511);
#9745=VERTEX_POINT('',#32513);
#9746=VERTEX_POINT('',#32517);
#9747=VERTEX_POINT('',#32523);
#9748=VERTEX_POINT('',#32525);
#9749=VERTEX_POINT('',#32529);
#9750=VERTEX_POINT('',#32535);
#9751=VERTEX_POINT('',#32537);
#9752=VERTEX_POINT('',#32541);
#9753=VERTEX_POINT('',#32547);
#9754=VERTEX_POINT('',#32551);
#9755=VERTEX_POINT('',#32555);
#9756=VERTEX_POINT('',#32559);
#9757=VERTEX_POINT('',#32563);
#9758=VERTEX_POINT('',#32567);
#9759=VERTEX_POINT('',#32571);
#9760=VERTEX_POINT('',#32573);
#9761=VERTEX_POINT('',#32577);
#9762=VERTEX_POINT('',#32578);
#9763=VERTEX_POINT('',#32585);
#9764=VERTEX_POINT('',#32586);
#9765=VERTEX_POINT('',#32591);
#9766=VERTEX_POINT('',#32595);
#9767=VERTEX_POINT('',#32598);
#9768=VERTEX_POINT('',#32599);
#9769=VERTEX_POINT('',#32603);
#9770=VERTEX_POINT('',#32609);
#9771=VERTEX_POINT('',#32610);
#9772=VERTEX_POINT('',#32614);
#9773=VERTEX_POINT('',#32620);
#9774=VERTEX_POINT('',#32621);
#9775=VERTEX_POINT('',#32625);
#9776=VERTEX_POINT('',#32637);
#9777=VERTEX_POINT('',#32638);
#9778=VERTEX_POINT('',#32642);
#9779=VERTEX_POINT('',#32648);
#9780=VERTEX_POINT('',#32649);
#9781=VERTEX_POINT('',#32653);
#9782=VERTEX_POINT('',#32659);
#9783=VERTEX_POINT('',#32660);
#9784=VERTEX_POINT('',#32664);
#11922=EDGE_CURVE('',#9662,#9663,#5975,.T.);
#11923=EDGE_CURVE('',#9663,#9664,#5976,.T.);
#11924=EDGE_CURVE('',#9664,#9665,#5977,.T.);
#11925=EDGE_CURVE('',#9665,#9662,#5978,.T.);
#11926=EDGE_CURVE('',#9663,#9666,#5979,.T.);
#11927=EDGE_CURVE('',#9666,#9667,#5980,.T.);
#11928=EDGE_CURVE('',#9667,#9664,#5981,.T.);
#11929=EDGE_CURVE('',#9668,#9669,#5982,.T.);
#11930=EDGE_CURVE('',#9669,#9667,#5151,.T.);
#11931=EDGE_CURVE('',#9666,#9668,#5152,.T.);
#11932=EDGE_CURVE('',#9670,#9671,#5983,.T.);
#11933=EDGE_CURVE('',#9671,#9669,#5984,.T.);
#11934=EDGE_CURVE('',#9668,#9670,#5985,.T.);
#11935=EDGE_CURVE('',#9672,#9673,#5986,.T.);
#11936=EDGE_CURVE('',#9673,#9671,#5153,.T.);
#11937=EDGE_CURVE('',#9670,#9672,#5154,.T.);
#11938=EDGE_CURVE('',#9665,#9673,#5987,.T.);
#11939=EDGE_CURVE('',#9672,#9662,#5988,.T.);
#11940=EDGE_CURVE('',#9674,#9673,#5989,.T.);
#11941=EDGE_CURVE('',#9675,#9674,#5155,.T.);
#11942=EDGE_CURVE('',#9675,#9671,#5990,.T.);
#11943=EDGE_CURVE('',#9665,#9676,#5991,.T.);
#11944=EDGE_CURVE('',#9674,#9676,#5992,.T.);
#11945=EDGE_CURVE('',#9664,#9677,#5993,.T.);
#11946=EDGE_CURVE('',#9676,#9677,#5994,.T.);
#11947=EDGE_CURVE('',#9678,#9678,#5156,.T.);
#11948=EDGE_CURVE('',#9679,#9679,#5157,.T.);
#11949=EDGE_CURVE('',#9680,#9680,#5158,.T.);
#11950=EDGE_CURVE('',#9681,#9681,#5159,.T.);
#11951=EDGE_CURVE('',#9682,#9682,#5160,.T.);
#11952=EDGE_CURVE('',#9683,#9683,#5161,.T.);
#11953=EDGE_CURVE('',#9684,#9684,#5162,.T.);
#11954=EDGE_CURVE('',#9685,#9676,#5995,.T.);
#11955=EDGE_CURVE('',#9677,#9686,#5996,.T.);
#11956=EDGE_CURVE('',#9686,#9687,#5997,.T.);
#11957=EDGE_CURVE('',#9687,#9688,#5998,.T.);
#11958=EDGE_CURVE('',#9688,#9685,#5999,.T.);
#11959=EDGE_CURVE('',#9689,#9687,#6000,.T.);
#11960=EDGE_CURVE('',#9690,#9689,#6001,.T.);
#11961=EDGE_CURVE('',#9688,#9690,#6002,.T.);
#11962=EDGE_CURVE('',#9691,#9691,#5163,.T.);
#11963=EDGE_CURVE('',#9692,#9692,#5164,.T.);
#11964=EDGE_CURVE('',#9693,#9693,#5165,.T.);
#11965=EDGE_CURVE('',#9694,#9686,#6003,.T.);
#11966=EDGE_CURVE('',#9694,#9695,#6004,.T.);
#11967=EDGE_CURVE('',#9695,#9696,#6005,.T.);
#11968=EDGE_CURVE('',#9696,#9689,#6006,.T.);
#11969=EDGE_CURVE('',#9677,#9697,#6007,.T.);
#11970=EDGE_CURVE('',#9698,#9697,#6008,.T.);
#11971=EDGE_CURVE('',#9698,#9694,#6009,.T.);
#11972=EDGE_CURVE('',#9685,#9699,#6010,.T.);
#11973=EDGE_CURVE('',#9699,#9700,#6011,.T.);
#11974=EDGE_CURVE('',#9700,#9674,#6012,.T.);
#11975=EDGE_CURVE('',#9701,#9675,#6013,.T.);
#11976=EDGE_CURVE('',#9700,#9701,#5166,.T.);
#11977=EDGE_CURVE('',#9702,#9703,#6014,.T.);
#11978=EDGE_CURVE('',#9703,#9675,#6015,.T.);
#11979=EDGE_CURVE('',#9701,#9702,#6016,.T.);
#11980=EDGE_CURVE('',#9697,#9703,#5167,.T.);
#11981=EDGE_CURVE('',#9702,#9698,#5168,.T.);
#11982=EDGE_CURVE('',#9703,#9669,#6017,.T.);
#11983=EDGE_CURVE('',#9697,#9667,#6018,.T.);
#11984=EDGE_CURVE('',#9696,#9704,#6019,.T.);
#11985=EDGE_CURVE('',#9704,#9705,#6020,.T.);
#11986=EDGE_CURVE('',#9705,#9706,#6021,.T.);
#11987=EDGE_CURVE('',#9690,#9706,#6022,.T.);
#11988=EDGE_CURVE('',#9706,#9707,#6023,.T.);
#11989=EDGE_CURVE('',#9707,#9699,#6024,.T.);
#11990=EDGE_CURVE('',#9708,#9707,#6025,.T.);
#11991=EDGE_CURVE('',#9700,#9708,#6026,.T.);
#11992=EDGE_CURVE('',#9705,#9709,#6027,.T.);
#11993=EDGE_CURVE('',#9708,#9709,#6028,.T.);
#11994=EDGE_CURVE('',#9695,#9710,#6029,.T.);
#11995=EDGE_CURVE('',#9710,#9711,#6030,.T.);
#11996=EDGE_CURVE('',#9711,#9704,#6031,.T.);
#11997=EDGE_CURVE('',#9712,#9713,#6032,.T.);
#11998=EDGE_CURVE('',#9713,#9711,#5169,.T.);
#11999=EDGE_CURVE('',#9710,#9712,#5170,.T.);
#12000=EDGE_CURVE('',#9714,#9715,#6033,.T.);
#12001=EDGE_CURVE('',#9715,#9713,#6034,.T.);
#12002=EDGE_CURVE('',#9712,#9714,#6035,.T.);
#12003=EDGE_CURVE('',#9709,#9715,#5171,.T.);
#12004=EDGE_CURVE('',#9714,#9708,#5172,.T.);
#12005=EDGE_CURVE('',#9709,#9716,#6036,.T.);
#12006=EDGE_CURVE('',#9717,#9716,#5173,.T.);
#12007=EDGE_CURVE('',#9715,#9717,#6037,.T.);
#12008=EDGE_CURVE('',#9718,#9705,#6038,.T.);
#12009=EDGE_CURVE('',#9716,#9718,#6039,.T.);
#12010=EDGE_CURVE('',#9719,#9704,#6040,.T.);
#12011=EDGE_CURVE('',#9718,#9719,#6041,.T.);
#12012=EDGE_CURVE('',#9702,#9712,#6042,.T.);
#12013=EDGE_CURVE('',#9710,#9698,#6043,.T.);
#12014=EDGE_CURVE('',#9720,#9721,#6044,.T.);
#12015=EDGE_CURVE('',#9721,#9718,#6045,.T.);
#12016=EDGE_CURVE('',#9719,#9720,#6046,.T.);
#12017=EDGE_CURVE('',#9721,#9722,#6047,.T.);
#12018=EDGE_CURVE('',#9722,#9716,#6048,.T.);
#12019=EDGE_CURVE('',#9723,#9717,#6049,.T.);
#12020=EDGE_CURVE('',#9722,#9723,#5174,.T.);
#12021=EDGE_CURVE('',#9724,#9725,#6050,.T.);
#12022=EDGE_CURVE('',#9725,#9717,#6051,.T.);
#12023=EDGE_CURVE('',#9723,#9724,#6052,.T.);
#12024=EDGE_CURVE('',#9726,#9727,#6053,.T.);
#12025=EDGE_CURVE('',#9727,#9725,#5175,.T.);
#12026=EDGE_CURVE('',#9724,#9726,#5176,.T.);
#12027=EDGE_CURVE('',#9719,#9727,#6054,.T.);
#12028=EDGE_CURVE('',#9726,#9720,#6055,.T.);
#12029=EDGE_CURVE('',#9713,#9725,#6056,.T.);
#12030=EDGE_CURVE('',#9711,#9727,#6057,.T.);
#12031=EDGE_CURVE('',#9728,#9728,#5177,.T.);
#12032=EDGE_CURVE('',#9729,#9729,#5178,.T.);
#12033=EDGE_CURVE('',#9730,#9730,#5179,.T.);
#12034=EDGE_CURVE('',#9731,#9731,#5180,.T.);
#12035=EDGE_CURVE('',#9732,#9732,#5181,.T.);
#12036=EDGE_CURVE('',#9733,#9733,#5182,.T.);
#12037=EDGE_CURVE('',#9734,#9734,#5183,.T.);
#12038=EDGE_CURVE('',#9735,#9735,#5184,.T.);
#12039=EDGE_CURVE('',#9736,#9736,#5185,.T.);
#12040=EDGE_CURVE('',#9737,#9737,#5186,.T.);
#12041=EDGE_CURVE('',#9678,#9738,#6058,.T.);
#12042=EDGE_CURVE('',#9738,#9738,#5187,.T.);
#12043=EDGE_CURVE('',#9738,#9739,#6059,.T.);
#12044=EDGE_CURVE('',#9739,#9739,#5188,.T.);
#12045=EDGE_CURVE('',#9728,#9740,#6060,.T.);
#12046=EDGE_CURVE('',#9740,#9741,#5189,.T.);
#12047=EDGE_CURVE('',#9741,#9740,#5190,.T.);
#12048=EDGE_CURVE('',#9742,#9742,#5191,.T.);
#12049=EDGE_CURVE('',#9742,#9741,#6061,.T.);
#12050=EDGE_CURVE('',#9739,#9743,#6062,.T.);
#12051=EDGE_CURVE('',#9743,#9743,#5192,.T.);
#12052=EDGE_CURVE('',#9737,#9744,#6063,.T.);
#12053=EDGE_CURVE('',#9744,#9745,#5193,.T.);
#12054=EDGE_CURVE('',#9745,#9744,#5194,.T.);
#12055=EDGE_CURVE('',#9746,#9746,#5195,.T.);
#12056=EDGE_CURVE('',#9746,#9745,#6064,.T.);
#12057=EDGE_CURVE('',#9684,#9746,#6065,.T.);
#12058=EDGE_CURVE('',#9729,#9747,#6066,.T.);
#12059=EDGE_CURVE('',#9747,#9748,#5196,.T.);
#12060=EDGE_CURVE('',#9748,#9747,#5197,.T.);
#12061=EDGE_CURVE('',#9749,#9749,#5198,.T.);
#12062=EDGE_CURVE('',#9749,#9748,#6067,.T.);
#12063=EDGE_CURVE('',#9679,#9749,#6068,.T.);
#12064=EDGE_CURVE('',#9736,#9750,#6069,.T.);
#12065=EDGE_CURVE('',#9750,#9751,#5199,.T.);
#12066=EDGE_CURVE('',#9751,#9750,#5200,.T.);
#12067=EDGE_CURVE('',#9752,#9752,#5201,.T.);
#12068=EDGE_CURVE('',#9752,#9751,#6070,.T.);
#12069=EDGE_CURVE('',#9683,#9752,#6071,.T.);
#12070=EDGE_CURVE('',#9680,#9753,#6072,.T.);
#12071=EDGE_CURVE('',#9753,#9753,#5202,.T.);
#12072=EDGE_CURVE('',#9753,#9754,#6073,.T.);
#12073=EDGE_CURVE('',#9754,#9754,#5203,.T.);
#12074=EDGE_CURVE('',#9682,#9755,#6074,.T.);
#12075=EDGE_CURVE('',#9755,#9755,#5204,.T.);
#12076=EDGE_CURVE('',#9755,#9756,#6075,.T.);
#12077=EDGE_CURVE('',#9756,#9756,#5205,.T.);
#12078=EDGE_CURVE('',#9681,#9757,#6076,.T.);
#12079=EDGE_CURVE('',#9757,#9757,#5206,.T.);
#12080=EDGE_CURVE('',#9757,#9758,#6077,.T.);
#12081=EDGE_CURVE('',#9758,#9758,#5207,.T.);
#12082=EDGE_CURVE('',#9759,#9759,#5208,.T.);
#12083=EDGE_CURVE('',#9759,#9760,#6078,.T.);
#12084=EDGE_CURVE('',#9760,#9760,#5209,.T.);
#12085=EDGE_CURVE('',#9761,#9762,#5210,.T.);
#12086=EDGE_CURVE('',#9762,#9761,#5211,.T.);
#12087=EDGE_CURVE('',#9762,#9760,#6079,.T.);
#12088=EDGE_CURVE('',#9714,#9701,#6080,.T.);
#12089=EDGE_CURVE('',#9763,#9764,#5212,.T.);
#12090=EDGE_CURVE('',#9764,#9763,#5213,.T.);
#12091=EDGE_CURVE('',#9763,#9761,#6081,.T.);
#12092=EDGE_CURVE('',#9765,#9765,#5214,.T.);
#12093=EDGE_CURVE('',#9765,#9764,#6082,.T.);
#12094=EDGE_CURVE('',#9766,#9765,#6083,.T.);
#12095=EDGE_CURVE('',#9767,#9768,#6084,.T.);
#12096=EDGE_CURVE('',#9768,#9768,#5215,.T.);
#12097=EDGE_CURVE('',#9768,#9769,#6085,.T.);
#12098=EDGE_CURVE('',#9769,#9769,#5216,.T.);
#12099=EDGE_CURVE('',#9769,#9693,#6086,.T.);
#12100=EDGE_CURVE('',#9770,#9771,#6087,.T.);
#12101=EDGE_CURVE('',#9771,#9771,#5217,.T.);
#12102=EDGE_CURVE('',#9771,#9772,#6088,.T.);
#12103=EDGE_CURVE('',#9772,#9772,#5218,.T.);
#12104=EDGE_CURVE('',#9772,#9692,#6089,.T.);
#12105=EDGE_CURVE('',#9773,#9774,#6090,.T.);
#12106=EDGE_CURVE('',#9774,#9774,#5219,.T.);
#12107=EDGE_CURVE('',#9774,#9775,#6091,.T.);
#12108=EDGE_CURVE('',#9775,#9775,#5220,.T.);
#12109=EDGE_CURVE('',#9775,#9691,#6092,.T.);
#12110=EDGE_CURVE('',#9758,#9730,#6093,.T.);
#12111=EDGE_CURVE('',#9756,#9735,#6094,.T.);
#12112=EDGE_CURVE('',#9754,#9731,#6095,.T.);
#12113=EDGE_CURVE('',#9776,#9777,#6096,.T.);
#12114=EDGE_CURVE('',#9777,#9777,#5221,.T.);
#12115=EDGE_CURVE('',#9777,#9778,#6097,.T.);
#12116=EDGE_CURVE('',#9778,#9778,#5222,.T.);
#12117=EDGE_CURVE('',#9778,#9732,#6098,.T.);
#12118=EDGE_CURVE('',#9779,#9780,#6099,.T.);
#12119=EDGE_CURVE('',#9780,#9780,#5223,.T.);
#12120=EDGE_CURVE('',#9780,#9781,#6100,.T.);
#12121=EDGE_CURVE('',#9781,#9781,#5224,.T.);
#12122=EDGE_CURVE('',#9781,#9733,#6101,.T.);
#12123=EDGE_CURVE('',#9782,#9783,#6102,.T.);
#12124=EDGE_CURVE('',#9783,#9783,#5225,.T.);
#12125=EDGE_CURVE('',#9783,#9784,#6103,.T.);
#12126=EDGE_CURVE('',#9784,#9784,#5226,.T.);
#12127=EDGE_CURVE('',#9784,#9734,#6104,.T.);
#15489=ORIENTED_EDGE('',*,*,#11922,.T.);
#15490=ORIENTED_EDGE('',*,*,#11923,.T.);
#15491=ORIENTED_EDGE('',*,*,#11924,.T.);
#15492=ORIENTED_EDGE('',*,*,#11925,.T.);
#15493=ORIENTED_EDGE('',*,*,#11926,.T.);
#15494=ORIENTED_EDGE('',*,*,#11927,.T.);
#15495=ORIENTED_EDGE('',*,*,#11928,.T.);
#15496=ORIENTED_EDGE('',*,*,#11923,.F.);
#15497=ORIENTED_EDGE('',*,*,#11929,.T.);
#15498=ORIENTED_EDGE('',*,*,#11930,.T.);
#15499=ORIENTED_EDGE('',*,*,#11927,.F.);
#15500=ORIENTED_EDGE('',*,*,#11931,.T.);
#15501=ORIENTED_EDGE('',*,*,#11932,.T.);
#15502=ORIENTED_EDGE('',*,*,#11933,.T.);
#15503=ORIENTED_EDGE('',*,*,#11929,.F.);
#15504=ORIENTED_EDGE('',*,*,#11934,.T.);
#15505=ORIENTED_EDGE('',*,*,#11935,.T.);
#15506=ORIENTED_EDGE('',*,*,#11936,.T.);
#15507=ORIENTED_EDGE('',*,*,#11932,.F.);
#15508=ORIENTED_EDGE('',*,*,#11937,.T.);
#15509=ORIENTED_EDGE('',*,*,#11938,.T.);
#15510=ORIENTED_EDGE('',*,*,#11935,.F.);
#15511=ORIENTED_EDGE('',*,*,#11939,.T.);
#15512=ORIENTED_EDGE('',*,*,#11925,.F.);
#15513=ORIENTED_EDGE('',*,*,#11936,.F.);
#15514=ORIENTED_EDGE('',*,*,#11940,.F.);
#15515=ORIENTED_EDGE('',*,*,#11941,.F.);
#15516=ORIENTED_EDGE('',*,*,#11942,.T.);
#15517=ORIENTED_EDGE('',*,*,#11938,.F.);
#15518=ORIENTED_EDGE('',*,*,#11943,.T.);
#15519=ORIENTED_EDGE('',*,*,#11944,.F.);
#15520=ORIENTED_EDGE('',*,*,#11940,.T.);
#15521=ORIENTED_EDGE('',*,*,#11924,.F.);
#15522=ORIENTED_EDGE('',*,*,#11945,.T.);
#15523=ORIENTED_EDGE('',*,*,#11946,.F.);
#15524=ORIENTED_EDGE('',*,*,#11943,.F.);
#15525=ORIENTED_EDGE('',*,*,#11922,.F.);
#15526=ORIENTED_EDGE('',*,*,#11939,.F.);
#15527=ORIENTED_EDGE('',*,*,#11937,.F.);
#15528=ORIENTED_EDGE('',*,*,#11934,.F.);
#15529=ORIENTED_EDGE('',*,*,#11931,.F.);
#15530=ORIENTED_EDGE('',*,*,#11926,.F.);
#15531=ORIENTED_EDGE('',*,*,#11947,.F.);
#15532=ORIENTED_EDGE('',*,*,#11948,.F.);
#15533=ORIENTED_EDGE('',*,*,#11949,.F.);
#15534=ORIENTED_EDGE('',*,*,#11950,.F.);
#15535=ORIENTED_EDGE('',*,*,#11951,.F.);
#15536=ORIENTED_EDGE('',*,*,#11952,.F.);
#15537=ORIENTED_EDGE('',*,*,#11953,.F.);
#15538=ORIENTED_EDGE('',*,*,#11954,.T.);
#15539=ORIENTED_EDGE('',*,*,#11946,.T.);
#15540=ORIENTED_EDGE('',*,*,#11955,.T.);
#15541=ORIENTED_EDGE('',*,*,#11956,.T.);
#15542=ORIENTED_EDGE('',*,*,#11957,.T.);
#15543=ORIENTED_EDGE('',*,*,#11958,.T.);
#15544=ORIENTED_EDGE('',*,*,#11957,.F.);
#15545=ORIENTED_EDGE('',*,*,#11959,.F.);
#15546=ORIENTED_EDGE('',*,*,#11960,.F.);
#15547=ORIENTED_EDGE('',*,*,#11961,.F.);
#15548=ORIENTED_EDGE('',*,*,#11962,.T.);
#15549=ORIENTED_EDGE('',*,*,#11963,.T.);
#15550=ORIENTED_EDGE('',*,*,#11964,.T.);
#15551=ORIENTED_EDGE('',*,*,#11956,.F.);
#15552=ORIENTED_EDGE('',*,*,#11965,.F.);
#15553=ORIENTED_EDGE('',*,*,#11966,.T.);
#15554=ORIENTED_EDGE('',*,*,#11967,.T.);
#15555=ORIENTED_EDGE('',*,*,#11968,.T.);
#15556=ORIENTED_EDGE('',*,*,#11959,.T.);
#15557=ORIENTED_EDGE('',*,*,#11955,.F.);
#15558=ORIENTED_EDGE('',*,*,#11969,.T.);
#15559=ORIENTED_EDGE('',*,*,#11970,.F.);
#15560=ORIENTED_EDGE('',*,*,#11971,.T.);
#15561=ORIENTED_EDGE('',*,*,#11965,.T.);
#15562=ORIENTED_EDGE('',*,*,#11954,.F.);
#15563=ORIENTED_EDGE('',*,*,#11972,.T.);
#15564=ORIENTED_EDGE('',*,*,#11973,.T.);
#15565=ORIENTED_EDGE('',*,*,#11974,.T.);
#15566=ORIENTED_EDGE('',*,*,#11944,.T.);
#15567=ORIENTED_EDGE('',*,*,#11975,.T.);
#15568=ORIENTED_EDGE('',*,*,#11941,.T.);
#15569=ORIENTED_EDGE('',*,*,#11974,.F.);
#15570=ORIENTED_EDGE('',*,*,#11976,.T.);
#15571=ORIENTED_EDGE('',*,*,#11977,.T.);
#15572=ORIENTED_EDGE('',*,*,#11978,.T.);
#15573=ORIENTED_EDGE('',*,*,#11975,.F.);
#15574=ORIENTED_EDGE('',*,*,#11979,.T.);
#15575=ORIENTED_EDGE('',*,*,#11970,.T.);
#15576=ORIENTED_EDGE('',*,*,#11980,.T.);
#15577=ORIENTED_EDGE('',*,*,#11977,.F.);
#15578=ORIENTED_EDGE('',*,*,#11981,.T.);
#15579=ORIENTED_EDGE('',*,*,#11933,.F.);
#15580=ORIENTED_EDGE('',*,*,#11942,.F.);
#15581=ORIENTED_EDGE('',*,*,#11978,.F.);
#15582=ORIENTED_EDGE('',*,*,#11982,.T.);
#15583=ORIENTED_EDGE('',*,*,#11930,.F.);
#15584=ORIENTED_EDGE('',*,*,#11982,.F.);
#15585=ORIENTED_EDGE('',*,*,#11980,.F.);
#15586=ORIENTED_EDGE('',*,*,#11983,.T.);
#15587=ORIENTED_EDGE('',*,*,#11928,.F.);
#15588=ORIENTED_EDGE('',*,*,#11983,.F.);
#15589=ORIENTED_EDGE('',*,*,#11969,.F.);
#15590=ORIENTED_EDGE('',*,*,#11945,.F.);
#15591=ORIENTED_EDGE('',*,*,#11968,.F.);
#15592=ORIENTED_EDGE('',*,*,#11984,.T.);
#15593=ORIENTED_EDGE('',*,*,#11985,.T.);
#15594=ORIENTED_EDGE('',*,*,#11986,.T.);
#15595=ORIENTED_EDGE('',*,*,#11987,.F.);
#15596=ORIENTED_EDGE('',*,*,#11960,.T.);
#15597=ORIENTED_EDGE('',*,*,#11958,.F.);
#15598=ORIENTED_EDGE('',*,*,#11961,.T.);
#15599=ORIENTED_EDGE('',*,*,#11987,.T.);
#15600=ORIENTED_EDGE('',*,*,#11988,.T.);
#15601=ORIENTED_EDGE('',*,*,#11989,.T.);
#15602=ORIENTED_EDGE('',*,*,#11972,.F.);
#15603=ORIENTED_EDGE('',*,*,#11973,.F.);
#15604=ORIENTED_EDGE('',*,*,#11989,.F.);
#15605=ORIENTED_EDGE('',*,*,#11990,.F.);
#15606=ORIENTED_EDGE('',*,*,#11991,.F.);
#15607=ORIENTED_EDGE('',*,*,#11988,.F.);
#15608=ORIENTED_EDGE('',*,*,#11986,.F.);
#15609=ORIENTED_EDGE('',*,*,#11992,.T.);
#15610=ORIENTED_EDGE('',*,*,#11993,.F.);
#15611=ORIENTED_EDGE('',*,*,#11990,.T.);
#15612=ORIENTED_EDGE('',*,*,#11967,.F.);
#15613=ORIENTED_EDGE('',*,*,#11994,.T.);
#15614=ORIENTED_EDGE('',*,*,#11995,.T.);
#15615=ORIENTED_EDGE('',*,*,#11996,.T.);
#15616=ORIENTED_EDGE('',*,*,#11984,.F.);
#15617=ORIENTED_EDGE('',*,*,#11997,.T.);
#15618=ORIENTED_EDGE('',*,*,#11998,.T.);
#15619=ORIENTED_EDGE('',*,*,#11995,.F.);
#15620=ORIENTED_EDGE('',*,*,#11999,.T.);
#15621=ORIENTED_EDGE('',*,*,#12000,.T.);
#15622=ORIENTED_EDGE('',*,*,#12001,.T.);
#15623=ORIENTED_EDGE('',*,*,#11997,.F.);
#15624=ORIENTED_EDGE('',*,*,#12002,.T.);
#15625=ORIENTED_EDGE('',*,*,#11993,.T.);
#15626=ORIENTED_EDGE('',*,*,#12003,.T.);
#15627=ORIENTED_EDGE('',*,*,#12000,.F.);
#15628=ORIENTED_EDGE('',*,*,#12004,.T.);
#15629=ORIENTED_EDGE('',*,*,#12003,.F.);
#15630=ORIENTED_EDGE('',*,*,#12005,.T.);
#15631=ORIENTED_EDGE('',*,*,#12006,.F.);
#15632=ORIENTED_EDGE('',*,*,#12007,.F.);
#15633=ORIENTED_EDGE('',*,*,#11992,.F.);
#15634=ORIENTED_EDGE('',*,*,#12008,.F.);
#15635=ORIENTED_EDGE('',*,*,#12009,.F.);
#15636=ORIENTED_EDGE('',*,*,#12005,.F.);
#15637=ORIENTED_EDGE('',*,*,#11985,.F.);
#15638=ORIENTED_EDGE('',*,*,#12010,.F.);
#15639=ORIENTED_EDGE('',*,*,#12011,.F.);
#15640=ORIENTED_EDGE('',*,*,#12008,.T.);
#15641=ORIENTED_EDGE('',*,*,#11981,.F.);
#15642=ORIENTED_EDGE('',*,*,#12012,.T.);
#15643=ORIENTED_EDGE('',*,*,#11999,.F.);
#15644=ORIENTED_EDGE('',*,*,#12013,.T.);
#15645=ORIENTED_EDGE('',*,*,#11971,.F.);
#15646=ORIENTED_EDGE('',*,*,#12013,.F.);
#15647=ORIENTED_EDGE('',*,*,#11994,.F.);
#15648=ORIENTED_EDGE('',*,*,#11966,.F.);
#15649=ORIENTED_EDGE('',*,*,#12014,.T.);
#15650=ORIENTED_EDGE('',*,*,#12015,.T.);
#15651=ORIENTED_EDGE('',*,*,#12011,.T.);
#15652=ORIENTED_EDGE('',*,*,#12016,.T.);
#15653=ORIENTED_EDGE('',*,*,#12017,.T.);
#15654=ORIENTED_EDGE('',*,*,#12018,.T.);
#15655=ORIENTED_EDGE('',*,*,#12009,.T.);
#15656=ORIENTED_EDGE('',*,*,#12015,.F.);
#15657=ORIENTED_EDGE('',*,*,#12019,.T.);
#15658=ORIENTED_EDGE('',*,*,#12006,.T.);
#15659=ORIENTED_EDGE('',*,*,#12018,.F.);
#15660=ORIENTED_EDGE('',*,*,#12020,.T.);
#15661=ORIENTED_EDGE('',*,*,#12021,.T.);
#15662=ORIENTED_EDGE('',*,*,#12022,.T.);
#15663=ORIENTED_EDGE('',*,*,#12019,.F.);
#15664=ORIENTED_EDGE('',*,*,#12023,.T.);
#15665=ORIENTED_EDGE('',*,*,#12024,.T.);
#15666=ORIENTED_EDGE('',*,*,#12025,.T.);
#15667=ORIENTED_EDGE('',*,*,#12021,.F.);
#15668=ORIENTED_EDGE('',*,*,#12026,.T.);
#15669=ORIENTED_EDGE('',*,*,#12027,.T.);
#15670=ORIENTED_EDGE('',*,*,#12024,.F.);
#15671=ORIENTED_EDGE('',*,*,#12028,.T.);
#15672=ORIENTED_EDGE('',*,*,#12016,.F.);
#15673=ORIENTED_EDGE('',*,*,#11998,.F.);
#15674=ORIENTED_EDGE('',*,*,#12029,.T.);
#15675=ORIENTED_EDGE('',*,*,#12025,.F.);
#15676=ORIENTED_EDGE('',*,*,#12030,.F.);
#15677=ORIENTED_EDGE('',*,*,#11996,.F.);
#15678=ORIENTED_EDGE('',*,*,#12030,.T.);
#15679=ORIENTED_EDGE('',*,*,#12027,.F.);
#15680=ORIENTED_EDGE('',*,*,#12010,.T.);
#15681=ORIENTED_EDGE('',*,*,#12014,.F.);
#15682=ORIENTED_EDGE('',*,*,#12028,.F.);
#15683=ORIENTED_EDGE('',*,*,#12026,.F.);
#15684=ORIENTED_EDGE('',*,*,#12023,.F.);
#15685=ORIENTED_EDGE('',*,*,#12020,.F.);
#15686=ORIENTED_EDGE('',*,*,#12017,.F.);
#15687=ORIENTED_EDGE('',*,*,#12031,.F.);
#15688=ORIENTED_EDGE('',*,*,#12032,.F.);
#15689=ORIENTED_EDGE('',*,*,#12033,.T.);
#15690=ORIENTED_EDGE('',*,*,#12034,.T.);
#15691=ORIENTED_EDGE('',*,*,#12035,.T.);
#15692=ORIENTED_EDGE('',*,*,#12036,.T.);
#15693=ORIENTED_EDGE('',*,*,#12037,.T.);
#15694=ORIENTED_EDGE('',*,*,#12038,.T.);
#15695=ORIENTED_EDGE('',*,*,#12039,.F.);
#15696=ORIENTED_EDGE('',*,*,#12040,.F.);
#15697=ORIENTED_EDGE('',*,*,#11947,.T.);
#15698=ORIENTED_EDGE('',*,*,#12041,.T.);
#15699=ORIENTED_EDGE('',*,*,#12042,.T.);
#15700=ORIENTED_EDGE('',*,*,#12041,.F.);
#15701=ORIENTED_EDGE('',*,*,#12042,.F.);
#15702=ORIENTED_EDGE('',*,*,#12043,.T.);
#15703=ORIENTED_EDGE('',*,*,#12044,.F.);
#15704=ORIENTED_EDGE('',*,*,#12043,.F.);
#15705=ORIENTED_EDGE('',*,*,#12031,.T.);
#15706=ORIENTED_EDGE('',*,*,#12045,.T.);
#15707=ORIENTED_EDGE('',*,*,#12046,.T.);
#15708=ORIENTED_EDGE('',*,*,#12047,.T.);
#15709=ORIENTED_EDGE('',*,*,#12045,.F.);
#15710=ORIENTED_EDGE('',*,*,#12048,.F.);
#15711=ORIENTED_EDGE('',*,*,#12049,.T.);
#15712=ORIENTED_EDGE('',*,*,#12046,.F.);
#15713=ORIENTED_EDGE('',*,*,#12047,.F.);
#15714=ORIENTED_EDGE('',*,*,#12049,.F.);
#15715=ORIENTED_EDGE('',*,*,#12044,.T.);
#15716=ORIENTED_EDGE('',*,*,#12050,.T.);
#15717=ORIENTED_EDGE('',*,*,#12051,.T.);
#15718=ORIENTED_EDGE('',*,*,#12050,.F.);
#15719=ORIENTED_EDGE('',*,*,#12048,.T.);
#15720=ORIENTED_EDGE('',*,*,#12051,.F.);
#15721=ORIENTED_EDGE('',*,*,#12040,.T.);
#15722=ORIENTED_EDGE('',*,*,#12052,.T.);
#15723=ORIENTED_EDGE('',*,*,#12053,.T.);
#15724=ORIENTED_EDGE('',*,*,#12054,.T.);
#15725=ORIENTED_EDGE('',*,*,#12052,.F.);
#15726=ORIENTED_EDGE('',*,*,#12055,.F.);
#15727=ORIENTED_EDGE('',*,*,#12056,.T.);
#15728=ORIENTED_EDGE('',*,*,#12053,.F.);
#15729=ORIENTED_EDGE('',*,*,#12054,.F.);
#15730=ORIENTED_EDGE('',*,*,#12056,.F.);
#15731=ORIENTED_EDGE('',*,*,#11953,.T.);
#15732=ORIENTED_EDGE('',*,*,#12057,.T.);
#15733=ORIENTED_EDGE('',*,*,#12055,.T.);
#15734=ORIENTED_EDGE('',*,*,#12057,.F.);
#15735=ORIENTED_EDGE('',*,*,#12032,.T.);
#15736=ORIENTED_EDGE('',*,*,#12058,.T.);
#15737=ORIENTED_EDGE('',*,*,#12059,.T.);
#15738=ORIENTED_EDGE('',*,*,#12060,.T.);
#15739=ORIENTED_EDGE('',*,*,#12058,.F.);
#15740=ORIENTED_EDGE('',*,*,#12061,.F.);
#15741=ORIENTED_EDGE('',*,*,#12062,.T.);
#15742=ORIENTED_EDGE('',*,*,#12059,.F.);
#15743=ORIENTED_EDGE('',*,*,#12060,.F.);
#15744=ORIENTED_EDGE('',*,*,#12062,.F.);
#15745=ORIENTED_EDGE('',*,*,#11948,.T.);
#15746=ORIENTED_EDGE('',*,*,#12063,.T.);
#15747=ORIENTED_EDGE('',*,*,#12061,.T.);
#15748=ORIENTED_EDGE('',*,*,#12063,.F.);
#15749=ORIENTED_EDGE('',*,*,#12039,.T.);
#15750=ORIENTED_EDGE('',*,*,#12064,.T.);
#15751=ORIENTED_EDGE('',*,*,#12065,.T.);
#15752=ORIENTED_EDGE('',*,*,#12066,.T.);
#15753=ORIENTED_EDGE('',*,*,#12064,.F.);
#15754=ORIENTED_EDGE('',*,*,#12067,.F.);
#15755=ORIENTED_EDGE('',*,*,#12068,.T.);
#15756=ORIENTED_EDGE('',*,*,#12065,.F.);
#15757=ORIENTED_EDGE('',*,*,#12066,.F.);
#15758=ORIENTED_EDGE('',*,*,#12068,.F.);
#15759=ORIENTED_EDGE('',*,*,#11952,.T.);
#15760=ORIENTED_EDGE('',*,*,#12069,.T.);
#15761=ORIENTED_EDGE('',*,*,#12067,.T.);
#15762=ORIENTED_EDGE('',*,*,#12069,.F.);
#15763=ORIENTED_EDGE('',*,*,#11949,.T.);
#15764=ORIENTED_EDGE('',*,*,#12070,.T.);
#15765=ORIENTED_EDGE('',*,*,#12071,.T.);
#15766=ORIENTED_EDGE('',*,*,#12070,.F.);
#15767=ORIENTED_EDGE('',*,*,#12071,.F.);
#15768=ORIENTED_EDGE('',*,*,#12072,.T.);
#15769=ORIENTED_EDGE('',*,*,#12073,.T.);
#15770=ORIENTED_EDGE('',*,*,#12072,.F.);
#15771=ORIENTED_EDGE('',*,*,#11951,.T.);
#15772=ORIENTED_EDGE('',*,*,#12074,.T.);
#15773=ORIENTED_EDGE('',*,*,#12075,.T.);
#15774=ORIENTED_EDGE('',*,*,#12074,.F.);
#15775=ORIENTED_EDGE('',*,*,#12075,.F.);
#15776=ORIENTED_EDGE('',*,*,#12076,.T.);
#15777=ORIENTED_EDGE('',*,*,#12077,.T.);
#15778=ORIENTED_EDGE('',*,*,#12076,.F.);
#15779=ORIENTED_EDGE('',*,*,#11950,.T.);
#15780=ORIENTED_EDGE('',*,*,#12078,.T.);
#15781=ORIENTED_EDGE('',*,*,#12079,.T.);
#15782=ORIENTED_EDGE('',*,*,#12078,.F.);
#15783=ORIENTED_EDGE('',*,*,#12079,.F.);
#15784=ORIENTED_EDGE('',*,*,#12080,.T.);
#15785=ORIENTED_EDGE('',*,*,#12081,.T.);
#15786=ORIENTED_EDGE('',*,*,#12080,.F.);
#15787=ORIENTED_EDGE('',*,*,#12082,.T.);
#15788=ORIENTED_EDGE('',*,*,#12083,.T.);
#15789=ORIENTED_EDGE('',*,*,#12084,.T.);
#15790=ORIENTED_EDGE('',*,*,#12083,.F.);
#15791=ORIENTED_EDGE('',*,*,#12085,.F.);
#15792=ORIENTED_EDGE('',*,*,#12086,.F.);
#15793=ORIENTED_EDGE('',*,*,#12087,.T.);
#15794=ORIENTED_EDGE('',*,*,#12084,.F.);
#15795=ORIENTED_EDGE('',*,*,#12087,.F.);
#15796=ORIENTED_EDGE('',*,*,#11979,.F.);
#15797=ORIENTED_EDGE('',*,*,#12088,.F.);
#15798=ORIENTED_EDGE('',*,*,#12002,.F.);
#15799=ORIENTED_EDGE('',*,*,#12012,.F.);
#15800=ORIENTED_EDGE('',*,*,#12082,.F.);
#15801=ORIENTED_EDGE('',*,*,#12089,.T.);
#15802=ORIENTED_EDGE('',*,*,#12090,.T.);
#15803=ORIENTED_EDGE('',*,*,#12091,.T.);
#15804=ORIENTED_EDGE('',*,*,#12085,.T.);
#15805=ORIENTED_EDGE('',*,*,#12086,.T.);
#15806=ORIENTED_EDGE('',*,*,#12091,.F.);
#15807=ORIENTED_EDGE('',*,*,#12092,.F.);
#15808=ORIENTED_EDGE('',*,*,#12093,.T.);
#15809=ORIENTED_EDGE('',*,*,#12089,.F.);
#15810=ORIENTED_EDGE('',*,*,#12090,.F.);
#15811=ORIENTED_EDGE('',*,*,#12093,.F.);
#15812=ORIENTED_EDGE('',*,*,#12094,.T.);
#15813=ORIENTED_EDGE('',*,*,#12092,.T.);
#15814=ORIENTED_EDGE('',*,*,#12094,.F.);
#15815=ORIENTED_EDGE('',*,*,#12095,.T.);
#15816=ORIENTED_EDGE('',*,*,#12096,.T.);
#15817=ORIENTED_EDGE('',*,*,#12095,.F.);
#15818=ORIENTED_EDGE('',*,*,#12096,.F.);
#15819=ORIENTED_EDGE('',*,*,#12097,.T.);
#15820=ORIENTED_EDGE('',*,*,#12098,.T.);
#15821=ORIENTED_EDGE('',*,*,#12097,.F.);
#15822=ORIENTED_EDGE('',*,*,#12098,.F.);
#15823=ORIENTED_EDGE('',*,*,#12099,.T.);
#15824=ORIENTED_EDGE('',*,*,#11964,.F.);
#15825=ORIENTED_EDGE('',*,*,#12099,.F.);
#15826=ORIENTED_EDGE('',*,*,#12100,.T.);
#15827=ORIENTED_EDGE('',*,*,#12101,.T.);
#15828=ORIENTED_EDGE('',*,*,#12100,.F.);
#15829=ORIENTED_EDGE('',*,*,#12101,.F.);
#15830=ORIENTED_EDGE('',*,*,#12102,.T.);
#15831=ORIENTED_EDGE('',*,*,#12103,.T.);
#15832=ORIENTED_EDGE('',*,*,#12102,.F.);
#15833=ORIENTED_EDGE('',*,*,#12103,.F.);
#15834=ORIENTED_EDGE('',*,*,#12104,.T.);
#15835=ORIENTED_EDGE('',*,*,#11963,.F.);
#15836=ORIENTED_EDGE('',*,*,#12104,.F.);
#15837=ORIENTED_EDGE('',*,*,#12105,.T.);
#15838=ORIENTED_EDGE('',*,*,#12106,.T.);
#15839=ORIENTED_EDGE('',*,*,#12105,.F.);
#15840=ORIENTED_EDGE('',*,*,#12106,.F.);
#15841=ORIENTED_EDGE('',*,*,#12107,.T.);
#15842=ORIENTED_EDGE('',*,*,#12108,.T.);
#15843=ORIENTED_EDGE('',*,*,#12107,.F.);
#15844=ORIENTED_EDGE('',*,*,#12108,.F.);
#15845=ORIENTED_EDGE('',*,*,#12109,.T.);
#15846=ORIENTED_EDGE('',*,*,#11962,.F.);
#15847=ORIENTED_EDGE('',*,*,#12109,.F.);
#15848=ORIENTED_EDGE('',*,*,#12081,.F.);
#15849=ORIENTED_EDGE('',*,*,#12110,.T.);
#15850=ORIENTED_EDGE('',*,*,#12033,.F.);
#15851=ORIENTED_EDGE('',*,*,#12110,.F.);
#15852=ORIENTED_EDGE('',*,*,#12077,.F.);
#15853=ORIENTED_EDGE('',*,*,#12111,.T.);
#15854=ORIENTED_EDGE('',*,*,#12038,.F.);
#15855=ORIENTED_EDGE('',*,*,#12111,.F.);
#15856=ORIENTED_EDGE('',*,*,#12073,.F.);
#15857=ORIENTED_EDGE('',*,*,#12112,.T.);
#15858=ORIENTED_EDGE('',*,*,#12034,.F.);
#15859=ORIENTED_EDGE('',*,*,#12112,.F.);
#15860=ORIENTED_EDGE('',*,*,#12113,.T.);
#15861=ORIENTED_EDGE('',*,*,#12114,.T.);
#15862=ORIENTED_EDGE('',*,*,#12113,.F.);
#15863=ORIENTED_EDGE('',*,*,#12114,.F.);
#15864=ORIENTED_EDGE('',*,*,#12115,.T.);
#15865=ORIENTED_EDGE('',*,*,#12116,.T.);
#15866=ORIENTED_EDGE('',*,*,#12115,.F.);
#15867=ORIENTED_EDGE('',*,*,#12116,.F.);
#15868=ORIENTED_EDGE('',*,*,#12117,.T.);
#15869=ORIENTED_EDGE('',*,*,#12035,.F.);
#15870=ORIENTED_EDGE('',*,*,#12117,.F.);
#15871=ORIENTED_EDGE('',*,*,#12118,.T.);
#15872=ORIENTED_EDGE('',*,*,#12119,.T.);
#15873=ORIENTED_EDGE('',*,*,#12118,.F.);
#15874=ORIENTED_EDGE('',*,*,#12119,.F.);
#15875=ORIENTED_EDGE('',*,*,#12120,.T.);
#15876=ORIENTED_EDGE('',*,*,#12121,.T.);
#15877=ORIENTED_EDGE('',*,*,#12120,.F.);
#15878=ORIENTED_EDGE('',*,*,#12121,.F.);
#15879=ORIENTED_EDGE('',*,*,#12122,.T.);
#15880=ORIENTED_EDGE('',*,*,#12036,.F.);
#15881=ORIENTED_EDGE('',*,*,#12122,.F.);
#15882=ORIENTED_EDGE('',*,*,#12123,.T.);
#15883=ORIENTED_EDGE('',*,*,#12124,.T.);
#15884=ORIENTED_EDGE('',*,*,#12123,.F.);
#15885=ORIENTED_EDGE('',*,*,#12124,.F.);
#15886=ORIENTED_EDGE('',*,*,#12125,.T.);
#15887=ORIENTED_EDGE('',*,*,#12126,.T.);
#15888=ORIENTED_EDGE('',*,*,#12125,.F.);
#15889=ORIENTED_EDGE('',*,*,#12126,.F.);
#15890=ORIENTED_EDGE('',*,*,#12127,.T.);
#15891=ORIENTED_EDGE('',*,*,#12037,.F.);
#15892=ORIENTED_EDGE('',*,*,#12127,.F.);
#15893=ORIENTED_EDGE('',*,*,#12001,.F.);
#15894=ORIENTED_EDGE('',*,*,#12007,.T.);
#15895=ORIENTED_EDGE('',*,*,#12022,.F.);
#15896=ORIENTED_EDGE('',*,*,#12029,.F.);
#15897=ORIENTED_EDGE('',*,*,#11976,.F.);
#15898=ORIENTED_EDGE('',*,*,#11991,.T.);
#15899=ORIENTED_EDGE('',*,*,#12004,.F.);
#15900=ORIENTED_EDGE('',*,*,#12088,.T.);
#21824=CONICAL_SURFACE('',#23689,0.515606601717798,1.17809724509616);
#21825=CONICAL_SURFACE('',#23693,0.515606601717797,1.17809724509619);
#21826=CONICAL_SURFACE('',#23697,0.56,0.785398163397454);
#21827=CONICAL_SURFACE('',#23717,0.589393398282201,0.392699081698744);
#21828=CONICAL_SURFACE('',#23720,0.589393398282202,0.39269908169875);
#21829=CONICAL_SURFACE('',#23724,0.56,0.785398163397454);
#21830=CONICAL_SURFACE('',#23731,0.589393398282202,0.392699081698749);
#21831=CONICAL_SURFACE('',#23735,0.589393398282201,0.392699081698732);
#21832=CONICAL_SURFACE('',#23738,0.56,0.785398163397454);
#21833=CONICAL_SURFACE('',#23746,0.515606601717797,1.17809724509618);
#21834=CONICAL_SURFACE('',#23749,0.515606601717798,1.17809724509616);
#21835=CONICAL_SURFACE('',#23753,0.56,0.785398163397454);
#21836=CONICAL_SURFACE('',#23766,3.315,0.785398163397444);
#21837=CONICAL_SURFACE('',#23770,3.79,0.785398163397448);
#21838=CONICAL_SURFACE('',#23775,3.315,0.785398163397444);
#21839=CONICAL_SURFACE('',#23778,0.185,0.785398163397448);
#21840=CONICAL_SURFACE('',#23783,0.185,0.785398163397444);
#21841=CONICAL_SURFACE('',#23784,0.185,0.785398163397456);
#21842=CONICAL_SURFACE('',#23789,0.185,0.785398163397452);
#21843=CONICAL_SURFACE('',#23790,0.185,0.785398163397448);
#21844=CONICAL_SURFACE('',#23795,0.185,0.785398163397444);
#21845=CONICAL_SURFACE('',#23796,0.42,0.785398163397452);
#21846=CONICAL_SURFACE('',#23800,0.419999999999999,0.785398163397452);
#21847=CONICAL_SURFACE('',#23804,0.42,0.785398163397447);
#21848=CONICAL_SURFACE('',#23808,0.459393398282203,1.17809724509617);
#21849=CONICAL_SURFACE('',#23811,0.455,0.785398163397442);
#21850=CONICAL_SURFACE('',#23815,0.415606601717798,0.392699081698719);
#21851=CONICAL_SURFACE('',#23820,0.2025,1.02974425867666);
#21852=CONICAL_SURFACE('',#23821,0.1275,1.02974425867665);
#21853=CONICAL_SURFACE('',#23825,0.305,0.785398163397446);
#21854=CONICAL_SURFACE('',#23826,0.1275,1.02974425867665);
#21855=CONICAL_SURFACE('',#23830,0.305,0.785398163397448);
#21856=CONICAL_SURFACE('',#23831,0.1275,1.02974425867665);
#21857=CONICAL_SURFACE('',#23835,0.305,0.785398163397446);
#21858=CONICAL_SURFACE('',#23836,0.43,0.558599315343562);
#21859=CONICAL_SURFACE('',#23837,0.429999999999999,0.558599315343561);
#21860=CONICAL_SURFACE('',#23838,0.430000000000001,0.558599315343561);
#21861=CONICAL_SURFACE('',#23839,0.0775000000000001,1.02974425867665);
#21862=CONICAL_SURFACE('',#23843,0.205,0.785398163397448);
#21863=CONICAL_SURFACE('',#23844,0.0775000000000001,1.02974425867665);
#21864=CONICAL_SURFACE('',#23848,0.205000000000001,0.785398163397448);
#21865=CONICAL_SURFACE('',#23849,0.0775000000000006,1.02974425867665);
#21866=CONICAL_SURFACE('',#23853,0.205,0.785398163397446);
#22075=ADVANCED_FACE('',(#2336),#1485,.T.);
#22076=ADVANCED_FACE('',(#2337),#1486,.T.);
#22077=ADVANCED_FACE('',(#2338),#21824,.T.);
#22078=ADVANCED_FACE('',(#2339),#1487,.T.);
#22079=ADVANCED_FACE('',(#2340),#21825,.T.);
#22080=ADVANCED_FACE('',(#2341),#1488,.T.);
#22081=ADVANCED_FACE('',(#2342),#21826,.T.);
#22082=ADVANCED_FACE('',(#2343),#1489,.T.);
#22083=ADVANCED_FACE('',(#2344),#1490,.T.);
#22084=ADVANCED_FACE('',(#2345,#1298,#1299,#1300,#1301,#1302,#1303,#1304),
#1491,.F.);
#22085=ADVANCED_FACE('',(#2346),#1492,.T.);
#22086=ADVANCED_FACE('',(#2347,#1305,#1306,#1307),#1493,.T.);
#22087=ADVANCED_FACE('',(#2348),#1494,.T.);
#22088=ADVANCED_FACE('',(#2349),#1495,.T.);
#22089=ADVANCED_FACE('',(#2350),#1496,.T.);
#22090=ADVANCED_FACE('',(#2351),#21827,.T.);
#22091=ADVANCED_FACE('',(#2352),#1497,.T.);
#22092=ADVANCED_FACE('',(#2353),#21828,.T.);
#22093=ADVANCED_FACE('',(#2354),#1498,.T.);
#22094=ADVANCED_FACE('',(#2355),#21829,.T.);
#22095=ADVANCED_FACE('',(#2356),#1499,.T.);
#22096=ADVANCED_FACE('',(#2357),#1500,.T.);
#22097=ADVANCED_FACE('',(#2358),#1501,.T.);
#22098=ADVANCED_FACE('',(#2359),#1502,.T.);
#22099=ADVANCED_FACE('',(#2360),#1503,.T.);
#22100=ADVANCED_FACE('',(#2361),#1504,.T.);
#22101=ADVANCED_FACE('',(#2362),#21830,.T.);
#22102=ADVANCED_FACE('',(#2363),#1505,.T.);
#22103=ADVANCED_FACE('',(#2364),#21831,.T.);
#22104=ADVANCED_FACE('',(#2365),#21832,.T.);
#22105=ADVANCED_FACE('',(#2366),#1506,.T.);
#22106=ADVANCED_FACE('',(#2367),#1507,.T.);
#22107=ADVANCED_FACE('',(#2368),#961,.T.);
#22108=ADVANCED_FACE('',(#2369),#1508,.T.);
#22109=ADVANCED_FACE('',(#2370),#1509,.T.);
#22110=ADVANCED_FACE('',(#2371),#1510,.T.);
#22111=ADVANCED_FACE('',(#2372),#21833,.T.);
#22112=ADVANCED_FACE('',(#2373),#1511,.T.);
#22113=ADVANCED_FACE('',(#2374),#21834,.T.);
#22114=ADVANCED_FACE('',(#2375),#1512,.T.);
#22115=ADVANCED_FACE('',(#2376),#21835,.T.);
#22116=ADVANCED_FACE('',(#2377),#1513,.T.);
#22117=ADVANCED_FACE('',(#2378,#1308,#1309,#1310,#1311,#1312,#1313,#1314,
#1315,#1316,#1317),#1514,.T.);
#22118=ADVANCED_FACE('',(#2379),#21836,.F.);
#22119=ADVANCED_FACE('',(#2380),#962,.F.);
#22120=ADVANCED_FACE('',(#2381),#21837,.F.);
#22121=ADVANCED_FACE('',(#2382),#963,.F.);
#22122=ADVANCED_FACE('',(#2383),#21838,.F.);
#22123=ADVANCED_FACE('',(#2384,#1318),#1515,.F.);
#22124=ADVANCED_FACE('',(#2385),#21839,.F.);
#22125=ADVANCED_FACE('',(#2386),#964,.F.);
#22126=ADVANCED_FACE('',(#2387),#21840,.F.);
#22127=ADVANCED_FACE('',(#2388),#21841,.F.);
#22128=ADVANCED_FACE('',(#2389),#965,.F.);
#22129=ADVANCED_FACE('',(#2390),#21842,.F.);
#22130=ADVANCED_FACE('',(#2391),#21843,.F.);
#22131=ADVANCED_FACE('',(#2392),#966,.F.);
#22132=ADVANCED_FACE('',(#2393),#21844,.F.);
#22133=ADVANCED_FACE('',(#2394),#21845,.F.);
#22134=ADVANCED_FACE('',(#2395),#967,.F.);
#22135=ADVANCED_FACE('',(#2396),#21846,.F.);
#22136=ADVANCED_FACE('',(#2397),#968,.F.);
#22137=ADVANCED_FACE('',(#2398),#21847,.F.);
#22138=ADVANCED_FACE('',(#2399),#969,.F.);
#22139=ADVANCED_FACE('',(#2400),#21848,.F.);
#22140=ADVANCED_FACE('',(#2401),#21849,.F.);
#22141=ADVANCED_FACE('',(#2402,#1319),#1516,.T.);
#22142=ADVANCED_FACE('',(#2403),#21850,.F.);
#22143=ADVANCED_FACE('',(#2404),#970,.F.);
#22144=ADVANCED_FACE('',(#2405),#21851,.F.);
#22145=ADVANCED_FACE('',(#2406),#21852,.F.);
#22146=ADVANCED_FACE('',(#2407),#971,.F.);
#22147=ADVANCED_FACE('',(#2408),#21853,.F.);
#22148=ADVANCED_FACE('',(#2409),#21854,.F.);
#22149=ADVANCED_FACE('',(#2410),#972,.F.);
#22150=ADVANCED_FACE('',(#2411),#21855,.F.);
#22151=ADVANCED_FACE('',(#2412),#21856,.F.);
#22152=ADVANCED_FACE('',(#2413),#973,.F.);
#22153=ADVANCED_FACE('',(#2414),#21857,.F.);
#22154=ADVANCED_FACE('',(#2415),#21858,.F.);
#22155=ADVANCED_FACE('',(#2416),#21859,.F.);
#22156=ADVANCED_FACE('',(#2417),#21860,.F.);
#22157=ADVANCED_FACE('',(#2418),#21861,.F.);
#22158=ADVANCED_FACE('',(#2419),#974,.F.);
#22159=ADVANCED_FACE('',(#2420),#21862,.F.);
#22160=ADVANCED_FACE('',(#2421),#21863,.F.);
#22161=ADVANCED_FACE('',(#2422),#975,.F.);
#22162=ADVANCED_FACE('',(#2423),#21864,.F.);
#22163=ADVANCED_FACE('',(#2424),#21865,.F.);
#22164=ADVANCED_FACE('',(#2425),#976,.F.);
#22165=ADVANCED_FACE('',(#2426),#21866,.F.);
#22166=ADVANCED_FACE('',(#2427),#1517,.T.);
#22167=ADVANCED_FACE('',(#2428),#977,.T.);
#23304=CLOSED_SHELL('',(#22075,#22076,#22077,#22078,#22079,#22080,#22081,
#22082,#22083,#22084,#22085,#22086,#22087,#22088,#22089,#22090,#22091,#22092,
#22093,#22094,#22095,#22096,#22097,#22098,#22099,#22100,#22101,#22102,#22103,
#22104,#22105,#22106,#22107,#22108,#22109,#22110,#22111,#22112,#22113,#22114,
#22115,#22116,#22117,#22118,#22119,#22120,#22121,#22122,#22123,#22124,#22125,
#22126,#22127,#22128,#22129,#22130,#22131,#22132,#22133,#22134,#22135,#22136,
#22137,#22138,#22139,#22140,#22141,#22142,#22143,#22144,#22145,#22146,#22147,
#22148,#22149,#22150,#22151,#22152,#22153,#22154,#22155,#22156,#22157,#22158,
#22159,#22160,#22161,#22162,#22163,#22164,#22165,#22166,#22167));
#23686=AXIS2_PLACEMENT_3D('',#32248,#26157,#26158);
#23687=AXIS2_PLACEMENT_3D('',#32249,#26159,#26160);
#23688=AXIS2_PLACEMENT_3D('',#32258,#26165,#26166);
#23689=AXIS2_PLACEMENT_3D('',#32264,#26170,#26171);
#23690=AXIS2_PLACEMENT_3D('',#32268,#26173,#26174);
#23691=AXIS2_PLACEMENT_3D('',#32269,#26175,#26176);
#23692=AXIS2_PLACEMENT_3D('',#32270,#26177,#26178);
#23693=AXIS2_PLACEMENT_3D('',#32276,#26182,#26183);
#23694=AXIS2_PLACEMENT_3D('',#32280,#26185,#26186);
#23695=AXIS2_PLACEMENT_3D('',#32281,#26187,#26188);
#23696=AXIS2_PLACEMENT_3D('',#32282,#26189,#26190);
#23697=AXIS2_PLACEMENT_3D('',#32285,#26193,#26194);
#23698=AXIS2_PLACEMENT_3D('',#32289,#26196,#26197);
#23699=AXIS2_PLACEMENT_3D('',#32291,#26199,#26200);
#23700=AXIS2_PLACEMENT_3D('',#32295,#26203,#26204);
#23701=AXIS2_PLACEMENT_3D('',#32299,#26207,#26208);
#23702=AXIS2_PLACEMENT_3D('',#32301,#26209,#26210);
#23703=AXIS2_PLACEMENT_3D('',#32303,#26211,#26212);
#23704=AXIS2_PLACEMENT_3D('',#32305,#26213,#26214);
#23705=AXIS2_PLACEMENT_3D('',#32307,#26215,#26216);
#23706=AXIS2_PLACEMENT_3D('',#32309,#26217,#26218);
#23707=AXIS2_PLACEMENT_3D('',#32311,#26219,#26220);
#23708=AXIS2_PLACEMENT_3D('',#32313,#26221,#26222);
#23709=AXIS2_PLACEMENT_3D('',#32314,#26223,#26224);
#23710=AXIS2_PLACEMENT_3D('',#32324,#26230,#26231);
#23711=AXIS2_PLACEMENT_3D('',#32331,#26235,#26236);
#23712=AXIS2_PLACEMENT_3D('',#32333,#26237,#26238);
#23713=AXIS2_PLACEMENT_3D('',#32335,#26239,#26240);
#23714=AXIS2_PLACEMENT_3D('',#32336,#26241,#26242);
#23715=AXIS2_PLACEMENT_3D('',#32344,#26247,#26248);
#23716=AXIS2_PLACEMENT_3D('',#32350,#26252,#26253);
#23717=AXIS2_PLACEMENT_3D('',#32356,#26257,#26258);
#23718=AXIS2_PLACEMENT_3D('',#32359,#26260,#26261);
#23719=AXIS2_PLACEMENT_3D('',#32360,#26262,#26263);
#23720=AXIS2_PLACEMENT_3D('',#32366,#26267,#26268);
#23721=AXIS2_PLACEMENT_3D('',#32367,#26269,#26270);
#23722=AXIS2_PLACEMENT_3D('',#32368,#26271,#26272);
#23723=AXIS2_PLACEMENT_3D('',#32369,#26273,#26274);
#23724=AXIS2_PLACEMENT_3D('',#32371,#26276,#26277);
#23725=AXIS2_PLACEMENT_3D('',#32373,#26279,#26280);
#23726=AXIS2_PLACEMENT_3D('',#32374,#26281,#26282);
#23727=AXIS2_PLACEMENT_3D('',#32382,#26287,#26288);
#23728=AXIS2_PLACEMENT_3D('',#32386,#26291,#26292);
#23729=AXIS2_PLACEMENT_3D('',#32390,#26295,#26296);
#23730=AXIS2_PLACEMENT_3D('',#32394,#26299,#26300);
#23731=AXIS2_PLACEMENT_3D('',#32400,#26304,#26305);
#23732=AXIS2_PLACEMENT_3D('',#32404,#26307,#26308);
#23733=AXIS2_PLACEMENT_3D('',#32405,#26309,#26310);
#23734=AXIS2_PLACEMENT_3D('',#32406,#26311,#26312);
#23735=AXIS2_PLACEMENT_3D('',#32412,#26316,#26317);
#23736=AXIS2_PLACEMENT_3D('',#32413,#26318,#26319);
#23737=AXIS2_PLACEMENT_3D('',#32414,#26320,#26321);
#23738=AXIS2_PLACEMENT_3D('',#32415,#26322,#26323);
#23739=AXIS2_PLACEMENT_3D('',#32419,#26325,#26326);
#23740=AXIS2_PLACEMENT_3D('',#32421,#26328,#26329);
#23741=AXIS2_PLACEMENT_3D('',#32425,#26332,#26333);
#23742=AXIS2_PLACEMENT_3D('',#32429,#26336,#26337);
#23743=AXIS2_PLACEMENT_3D('',#32432,#26340,#26341);
#23744=AXIS2_PLACEMENT_3D('',#32433,#26342,#26343);
#23745=AXIS2_PLACEMENT_3D('',#32439,#26347,#26348);
#23746=AXIS2_PLACEMENT_3D('',#32443,#26351,#26352);
#23747=AXIS2_PLACEMENT_3D('',#32446,#26354,#26355);
#23748=AXIS2_PLACEMENT_3D('',#32447,#26356,#26357);
#23749=AXIS2_PLACEMENT_3D('',#32453,#26361,#26362);
#23750=AXIS2_PLACEMENT_3D('',#32457,#26364,#26365);
#23751=AXIS2_PLACEMENT_3D('',#32458,#26366,#26367);
#23752=AXIS2_PLACEMENT_3D('',#32459,#26368,#26369);
#23753=AXIS2_PLACEMENT_3D('',#32462,#26372,#26373);
#23754=AXIS2_PLACEMENT_3D('',#32465,#26376,#26377);
#23755=AXIS2_PLACEMENT_3D('',#32466,#26378,#26379);
#23756=AXIS2_PLACEMENT_3D('',#32468,#26380,#26381);
#23757=AXIS2_PLACEMENT_3D('',#32470,#26382,#26383);
#23758=AXIS2_PLACEMENT_3D('',#32472,#26384,#26385);
#23759=AXIS2_PLACEMENT_3D('',#32474,#26386,#26387);
#23760=AXIS2_PLACEMENT_3D('',#32476,#26388,#26389);
#23761=AXIS2_PLACEMENT_3D('',#32478,#26390,#26391);
#23762=AXIS2_PLACEMENT_3D('',#32480,#26392,#26393);
#23763=AXIS2_PLACEMENT_3D('',#32482,#26394,#26395);
#23764=AXIS2_PLACEMENT_3D('',#32484,#26396,#26397);
#23765=AXIS2_PLACEMENT_3D('',#32486,#26398,#26399);
#23766=AXIS2_PLACEMENT_3D('',#32487,#26400,#26401);
#23767=AXIS2_PLACEMENT_3D('',#32490,#26403,#26404);
#23768=AXIS2_PLACEMENT_3D('',#32491,#26405,#26406);
#23769=AXIS2_PLACEMENT_3D('',#32494,#26408,#26409);
#23770=AXIS2_PLACEMENT_3D('',#32495,#26410,#26411);
#23771=AXIS2_PLACEMENT_3D('',#32499,#26413,#26414);
#23772=AXIS2_PLACEMENT_3D('',#32500,#26415,#26416);
#23773=AXIS2_PLACEMENT_3D('',#32501,#26417,#26418);
#23774=AXIS2_PLACEMENT_3D('',#32503,#26419,#26420);
#23775=AXIS2_PLACEMENT_3D('',#32505,#26422,#26423);
#23776=AXIS2_PLACEMENT_3D('',#32508,#26425,#26426);
#23777=AXIS2_PLACEMENT_3D('',#32509,#26427,#26428);
#23778=AXIS2_PLACEMENT_3D('',#32510,#26429,#26430);
#23779=AXIS2_PLACEMENT_3D('',#32514,#26432,#26433);
#23780=AXIS2_PLACEMENT_3D('',#32515,#26434,#26435);
#23781=AXIS2_PLACEMENT_3D('',#32516,#26436,#26437);
#23782=AXIS2_PLACEMENT_3D('',#32518,#26438,#26439);
#23783=AXIS2_PLACEMENT_3D('',#32520,#26441,#26442);
#23784=AXIS2_PLACEMENT_3D('',#32522,#26444,#26445);
#23785=AXIS2_PLACEMENT_3D('',#32526,#26447,#26448);
#23786=AXIS2_PLACEMENT_3D('',#32527,#26449,#26450);
#23787=AXIS2_PLACEMENT_3D('',#32528,#26451,#26452);
#23788=AXIS2_PLACEMENT_3D('',#32530,#26453,#26454);
#23789=AXIS2_PLACEMENT_3D('',#32532,#26456,#26457);
#23790=AXIS2_PLACEMENT_3D('',#32534,#26459,#26460);
#23791=AXIS2_PLACEMENT_3D('',#32538,#26462,#26463);
#23792=AXIS2_PLACEMENT_3D('',#32539,#26464,#26465);
#23793=AXIS2_PLACEMENT_3D('',#32540,#26466,#26467);
#23794=AXIS2_PLACEMENT_3D('',#32542,#26468,#26469);
#23795=AXIS2_PLACEMENT_3D('',#32544,#26471,#26472);
#23796=AXIS2_PLACEMENT_3D('',#32546,#26474,#26475);
#23797=AXIS2_PLACEMENT_3D('',#32549,#26477,#26478);
#23798=AXIS2_PLACEMENT_3D('',#32550,#26479,#26480);
#23799=AXIS2_PLACEMENT_3D('',#32553,#26482,#26483);
#23800=AXIS2_PLACEMENT_3D('',#32554,#26484,#26485);
#23801=AXIS2_PLACEMENT_3D('',#32557,#26487,#26488);
#23802=AXIS2_PLACEMENT_3D('',#32558,#26489,#26490);
#23803=AXIS2_PLACEMENT_3D('',#32561,#26492,#26493);
#23804=AXIS2_PLACEMENT_3D('',#32562,#26494,#26495);
#23805=AXIS2_PLACEMENT_3D('',#32565,#26497,#26498);
#23806=AXIS2_PLACEMENT_3D('',#32566,#26499,#26500);
#23807=AXIS2_PLACEMENT_3D('',#32569,#26502,#26503);
#23808=AXIS2_PLACEMENT_3D('',#32570,#26504,#26505);
#23809=AXIS2_PLACEMENT_3D('',#32572,#26506,#26507);
#23810=AXIS2_PLACEMENT_3D('',#32575,#26509,#26510);
#23811=AXIS2_PLACEMENT_3D('',#32576,#26511,#26512);
#23812=AXIS2_PLACEMENT_3D('',#32579,#26513,#26514);
#23813=AXIS2_PLACEMENT_3D('',#32580,#26515,#26516);
#23814=AXIS2_PLACEMENT_3D('',#32582,#26518,#26519);
#23815=AXIS2_PLACEMENT_3D('',#32584,#26521,#26522);
#23816=AXIS2_PLACEMENT_3D('',#32587,#26523,#26524);
#23817=AXIS2_PLACEMENT_3D('',#32588,#26525,#26526);
#23818=AXIS2_PLACEMENT_3D('',#32590,#26528,#26529);
#23819=AXIS2_PLACEMENT_3D('',#32592,#26530,#26531);
#23820=AXIS2_PLACEMENT_3D('',#32594,#26533,#26534);
#23821=AXIS2_PLACEMENT_3D('',#32597,#26536,#26537);
#23822=AXIS2_PLACEMENT_3D('',#32601,#26539,#26540);
#23823=AXIS2_PLACEMENT_3D('',#32602,#26541,#26542);
#23824=AXIS2_PLACEMENT_3D('',#32605,#26544,#26545);
#23825=AXIS2_PLACEMENT_3D('',#32606,#26546,#26547);
#23826=AXIS2_PLACEMENT_3D('',#32608,#26549,#26550);
#23827=AXIS2_PLACEMENT_3D('',#32612,#26552,#26553);
#23828=AXIS2_PLACEMENT_3D('',#32613,#26554,#26555);
#23829=AXIS2_PLACEMENT_3D('',#32616,#26557,#26558);
#23830=AXIS2_PLACEMENT_3D('',#32617,#26559,#26560);
#23831=AXIS2_PLACEMENT_3D('',#32619,#26562,#26563);
#23832=AXIS2_PLACEMENT_3D('',#32623,#26565,#26566);
#23833=AXIS2_PLACEMENT_3D('',#32624,#26567,#26568);
#23834=AXIS2_PLACEMENT_3D('',#32627,#26570,#26571);
#23835=AXIS2_PLACEMENT_3D('',#32628,#26572,#26573);
#23836=AXIS2_PLACEMENT_3D('',#32630,#26575,#26576);
#23837=AXIS2_PLACEMENT_3D('',#32632,#26578,#26579);
#23838=AXIS2_PLACEMENT_3D('',#32634,#26581,#26582);
#23839=AXIS2_PLACEMENT_3D('',#32636,#26584,#26585);
#23840=AXIS2_PLACEMENT_3D('',#32640,#26587,#26588);
#23841=AXIS2_PLACEMENT_3D('',#32641,#26589,#26590);
#23842=AXIS2_PLACEMENT_3D('',#32644,#26592,#26593);
#23843=AXIS2_PLACEMENT_3D('',#32645,#26594,#26595);
#23844=AXIS2_PLACEMENT_3D('',#32647,#26597,#26598);
#23845=AXIS2_PLACEMENT_3D('',#32651,#26600,#26601);
#23846=AXIS2_PLACEMENT_3D('',#32652,#26602,#26603);
#23847=AXIS2_PLACEMENT_3D('',#32655,#26605,#26606);
#23848=AXIS2_PLACEMENT_3D('',#32656,#26607,#26608);
#23849=AXIS2_PLACEMENT_3D('',#32658,#26610,#26611);
#23850=AXIS2_PLACEMENT_3D('',#32662,#26613,#26614);
#23851=AXIS2_PLACEMENT_3D('',#32663,#26615,#26616);
#23852=AXIS2_PLACEMENT_3D('',#32666,#26618,#26619);
#23853=AXIS2_PLACEMENT_3D('',#32667,#26620,#26621);
#23854=AXIS2_PLACEMENT_3D('',#32669,#26623,#26624);
#23855=AXIS2_PLACEMENT_3D('',#32670,#26625,#26626);
#26157=DIRECTION('axis',(0.,0.,1.));
#26158=DIRECTION('refdir',(1.,0.,0.));
#26159=DIRECTION('center_axis',(0.,-0.923879532511281,-0.382683432365103));
#26160=DIRECTION('ref_axis',(0.,0.382683432365103,-0.923879532511281));
#26161=DIRECTION('',(-1.,0.,0.));
#26162=DIRECTION('',(-0.678598344545856,0.281084637714825,-0.678598344545836));
#26163=DIRECTION('',(1.,0.,0.));
#26164=DIRECTION('',(-0.678598344545858,-0.281084637714826,0.678598344545834));
#26165=DIRECTION('center_axis',(-0.382683432365088,-0.923879532511288,0.));
#26166=DIRECTION('ref_axis',(0.,0.,-1.));
#26167=DIRECTION('',(0.,0.,1.));
#26168=DIRECTION('',(-0.923879532511283,0.3826834323651,0.));
#26169=DIRECTION('',(0.,0.,-1.));
#26170=DIRECTION('center_axis',(0.,1.,0.));
#26171=DIRECTION('ref_axis',(-0.707106781186549,0.,0.707106781186546));
#26172=DIRECTION('',(0.,0.382683432365092,0.923879532511286));
#26173=DIRECTION('center_axis',(-8.70318267579337E-16,-1.,-8.70318267579341E-16));
#26174=DIRECTION('ref_axis',(-0.707106781186549,0.,0.707106781186546));
#26175=DIRECTION('center_axis',(0.,1.,0.));
#26176=DIRECTION('ref_axis',(-0.70710678118655,0.,0.707106781186545));
#26177=DIRECTION('center_axis',(0.,-0.923879532511287,0.382683432365089));
#26178=DIRECTION('ref_axis',(0.,-0.382683432365089,-0.923879532511287));
#26179=DIRECTION('',(0.,0.382683432365109,0.923879532511279));
#26180=DIRECTION('',(-1.,0.,0.));
#26181=DIRECTION('',(1.,0.,0.));
#26182=DIRECTION('center_axis',(0.,1.,0.));
#26183=DIRECTION('ref_axis',(0.707106781186548,0.,0.707106781186548));
#26184=DIRECTION('',(0.923879532511298,0.382683432365064,0.));
#26185=DIRECTION('center_axis',(0.,-1.,0.));
#26186=DIRECTION('ref_axis',(0.707106781186548,0.,0.707106781186548));
#26187=DIRECTION('center_axis',(0.,1.,0.));
#26188=DIRECTION('ref_axis',(0.707106781186547,0.,0.707106781186547));
#26189=DIRECTION('center_axis',(0.382683432365088,-0.923879532511288,0.));
#26190=DIRECTION('ref_axis',(0.,0.,-1.));
#26191=DIRECTION('',(0.,0.,1.));
#26192=DIRECTION('',(0.,0.,-1.));
#26193=DIRECTION('center_axis',(0.,1.,0.));
#26194=DIRECTION('ref_axis',(0.707106781186548,0.,0.707106781186548));
#26195=DIRECTION('',(-0.707106781186548,-0.707106781186548,0.));
#26196=DIRECTION('center_axis',(0.,1.,0.));
#26197=DIRECTION('ref_axis',(0.707106781186548,0.,0.707106781186547));
#26198=DIRECTION('',(0.,-0.70710678118654,-0.707106781186555));
#26199=DIRECTION('center_axis',(0.707106781186548,-0.707106781186548,0.));
#26200=DIRECTION('ref_axis',(0.,0.,-1.));
#26201=DIRECTION('',(0.577350269189625,0.577350269189625,-0.577350269189627));
#26202=DIRECTION('',(0.,0.,-1.));
#26203=DIRECTION('center_axis',(0.,-0.707106781186549,-0.707106781186547));
#26204=DIRECTION('ref_axis',(-1.,0.,0.));
#26205=DIRECTION('',(-0.577350269189624,0.577350269189624,-0.57735026918963));
#26206=DIRECTION('',(-1.,0.,0.));
#26207=DIRECTION('center_axis',(0.,1.,0.));
#26208=DIRECTION('ref_axis',(1.,0.,0.));
#26209=DIRECTION('center_axis',(0.,-1.,0.));
#26210=DIRECTION('ref_axis',(-1.,0.,0.));
#26211=DIRECTION('center_axis',(0.,-1.,0.));
#26212=DIRECTION('ref_axis',(-1.,0.,0.));
#26213=DIRECTION('center_axis',(0.,-1.,0.));
#26214=DIRECTION('ref_axis',(-1.,0.,0.));
#26215=DIRECTION('center_axis',(0.,-1.,0.));
#26216=DIRECTION('ref_axis',(-1.,0.,0.));
#26217=DIRECTION('center_axis',(0.,-1.,0.));
#26218=DIRECTION('ref_axis',(-1.,0.,0.));
#26219=DIRECTION('center_axis',(0.,-1.,0.));
#26220=DIRECTION('ref_axis',(-1.,0.,0.));
#26221=DIRECTION('center_axis',(0.,-1.,0.));
#26222=DIRECTION('ref_axis',(-1.,0.,0.));
#26223=DIRECTION('center_axis',(0.,-0.382683432365092,-0.923879532511286));
#26224=DIRECTION('ref_axis',(-1.,0.,0.));
#26225=DIRECTION('',(-0.357406744336597,-0.862856209461015,0.357406744336595));
#26226=DIRECTION('',(-0.357406744336597,0.862856209461015,-0.357406744336595));
#26227=DIRECTION('',(0.357406744336602,0.862856209461013,-0.357406744336594));
#26228=DIRECTION('',(1.,0.,0.));
#26229=DIRECTION('',(0.357406744336593,-0.862856209461016,0.357406744336595));
#26230=DIRECTION('center_axis',(0.,0.,-1.));
#26231=DIRECTION('ref_axis',(-1.,0.,0.));
#26232=DIRECTION('',(0.,-1.,0.));
#26233=DIRECTION('',(-1.,0.,0.));
#26234=DIRECTION('',(0.,1.,0.));
#26235=DIRECTION('center_axis',(0.,0.,1.));
#26236=DIRECTION('ref_axis',(-1.,0.,0.));
#26237=DIRECTION('center_axis',(0.,0.,1.));
#26238=DIRECTION('ref_axis',(-1.,0.,0.));
#26239=DIRECTION('center_axis',(0.,0.,1.));
#26240=DIRECTION('ref_axis',(-1.,0.,0.));
#26241=DIRECTION('center_axis',(-0.70710678118654,0.,-0.707106781186555));
#26242=DIRECTION('ref_axis',(-0.707106781186555,0.,0.70710678118654));
#26243=DIRECTION('',(0.357406744336598,-0.862856209461016,-0.35740674433659));
#26244=DIRECTION('',(0.,1.,0.));
#26245=DIRECTION('',(0.3574067443366,0.862856209461015,-0.357406744336592));
#26246=DIRECTION('',(0.357406744336606,-0.86285620946101,-0.357406744336598));
#26247=DIRECTION('center_axis',(-0.923879532511285,-0.382683432365094,0.));
#26248=DIRECTION('ref_axis',(0.,0.,1.));
#26249=DIRECTION('',(0.,0.,1.));
#26250=DIRECTION('',(0.382683432365092,-0.923879532511286,0.));
#26251=DIRECTION('',(0.,0.,-1.));
#26252=DIRECTION('center_axis',(0.923879532511285,-0.382683432365094,0.));
#26253=DIRECTION('ref_axis',(0.,0.,-1.));
#26254=DIRECTION('',(0.357406744336596,0.862856209461013,0.357406744336599));
#26255=DIRECTION('',(0.,0.,1.));
#26256=DIRECTION('',(-0.382683432365095,-0.923879532511285,0.));
#26257=DIRECTION('center_axis',(0.,1.,0.));
#26258=DIRECTION('ref_axis',(0.707106781186548,0.,0.707106781186547));
#26259=DIRECTION('',(0.,-0.923879532511273,-0.382683432365123));
#26260=DIRECTION('center_axis',(0.,-1.,0.));
#26261=DIRECTION('ref_axis',(0.707106781186548,0.,0.707106781186548));
#26262=DIRECTION('center_axis',(0.,-0.382683432365085,0.923879532511289));
#26263=DIRECTION('ref_axis',(1.,0.,0.));
#26264=DIRECTION('',(0.,-0.92387953251129,-0.382683432365083));
#26265=DIRECTION('',(1.,0.,0.));
#26266=DIRECTION('',(-1.,0.,0.));
#26267=DIRECTION('center_axis',(0.,1.,3.46855248302154E-14));
#26268=DIRECTION('ref_axis',(-0.70710678118655,0.,0.707106781186545));
#26269=DIRECTION('center_axis',(-5.42546052537348E-16,1.,-5.42546052537352E-16));
#26270=DIRECTION('ref_axis',(-0.70710678118655,0.,0.707106781186545));
#26271=DIRECTION('center_axis',(0.,-1.,0.));
#26272=DIRECTION('ref_axis',(-0.70710678118655,0.,0.707106781186545));
#26273=DIRECTION('center_axis',(0.,-0.70710678118654,0.707106781186555));
#26274=DIRECTION('ref_axis',(1.,0.,0.));
#26275=DIRECTION('',(0.,-0.707106781186555,-0.70710678118654));
#26276=DIRECTION('center_axis',(0.,1.,0.));
#26277=DIRECTION('ref_axis',(-0.70710678118655,0.,0.707106781186545));
#26278=DIRECTION('',(0.707106781186551,-0.707106781186544,0.));
#26279=DIRECTION('center_axis',(-0.707106781186548,-0.707106781186548,0.));
#26280=DIRECTION('ref_axis',(0.,0.,1.));
#26281=DIRECTION('center_axis',(0.,0.382683432365097,-0.923879532511284));
#26282=DIRECTION('ref_axis',(-1.,0.,0.));
#26283=DIRECTION('',(0.357406744336598,0.86285620946101,0.357406744336605));
#26284=DIRECTION('',(1.,0.,0.));
#26285=DIRECTION('',(0.357406744336598,-0.862856209461011,-0.357406744336602));
#26286=DIRECTION('',(0.357406744336597,0.862856209461013,0.357406744336599));
#26287=DIRECTION('center_axis',(0.70710678118655,0.,-0.707106781186545));
#26288=DIRECTION('ref_axis',(-0.707106781186545,0.,-0.70710678118655));
#26289=DIRECTION('',(0.357406744336599,-0.862856209461011,0.357406744336601));
#26290=DIRECTION('',(0.,-1.,0.));
#26291=DIRECTION('center_axis',(1.,0.,0.));
#26292=DIRECTION('ref_axis',(0.,0.,-1.));
#26293=DIRECTION('',(0.,0.,-1.));
#26294=DIRECTION('',(0.,1.,0.));
#26295=DIRECTION('center_axis',(0.923879532511284,0.382683432365097,0.));
#26296=DIRECTION('ref_axis',(0.,0.,-1.));
#26297=DIRECTION('',(0.,0.,1.));
#26298=DIRECTION('',(-0.382683432365099,0.923879532511283,0.));
#26299=DIRECTION('center_axis',(-0.923879532511284,0.382683432365097,0.));
#26300=DIRECTION('ref_axis',(0.,0.,1.));
#26301=DIRECTION('',(0.,0.,1.));
#26302=DIRECTION('',(0.382683432365097,0.923879532511284,0.));
#26303=DIRECTION('',(0.,0.,-1.));
#26304=DIRECTION('center_axis',(0.,-1.,3.46855248302153E-14));
#26305=DIRECTION('ref_axis',(-0.70710678118655,0.,0.707106781186545));
#26306=DIRECTION('',(0.,0.923879532511285,-0.382683432365094));
#26307=DIRECTION('center_axis',(0.,-1.,0.));
#26308=DIRECTION('ref_axis',(-0.70710678118655,0.,0.707106781186545));
#26309=DIRECTION('center_axis',(0.,1.,0.));
#26310=DIRECTION('ref_axis',(-0.70710678118655,0.,0.707106781186545));
#26311=DIRECTION('center_axis',(0.,0.382683432365083,0.92387953251129));
#26312=DIRECTION('ref_axis',(1.,0.,0.));
#26313=DIRECTION('',(0.,0.923879532511292,-0.382683432365077));
#26314=DIRECTION('',(-1.,0.,0.));
#26315=DIRECTION('',(1.,0.,0.));
#26316=DIRECTION('center_axis',(0.,-1.,0.));
#26317=DIRECTION('ref_axis',(0.707106781186548,0.,0.707106781186547));
#26318=DIRECTION('center_axis',(0.,-1.,0.));
#26319=DIRECTION('ref_axis',(0.707106781186549,0.,0.707106781186546));
#26320=DIRECTION('center_axis',(0.,1.,0.));
#26321=DIRECTION('ref_axis',(0.707106781186547,0.,0.707106781186547));
#26322=DIRECTION('center_axis',(0.,-1.,0.));
#26323=DIRECTION('ref_axis',(0.707106781186548,0.,0.707106781186548));
#26324=DIRECTION('',(-0.707106781186551,0.707106781186544,0.));
#26325=DIRECTION('center_axis',(0.,1.,0.));
#26326=DIRECTION('ref_axis',(0.707106781186548,0.,0.707106781186548));
#26327=DIRECTION('',(0.,0.707106781186555,-0.70710678118654));
#26328=DIRECTION('center_axis',(0.707106781186548,0.707106781186548,0.));
#26329=DIRECTION('ref_axis',(0.,0.,-1.));
#26330=DIRECTION('',(0.577350269189623,-0.577350269189623,-0.577350269189631));
#26331=DIRECTION('',(0.,0.,-1.));
#26332=DIRECTION('center_axis',(0.,0.707106781186549,-0.707106781186547));
#26333=DIRECTION('ref_axis',(-1.,0.,0.));
#26334=DIRECTION('',(-0.577350269189619,-0.577350269189626,-0.577350269189632));
#26335=DIRECTION('',(-1.,0.,0.));
#26336=DIRECTION('center_axis',(0.,1.,0.));
#26337=DIRECTION('ref_axis',(-0.70710678118655,0.,0.707106781186545));
#26338=DIRECTION('',(0.,1.,0.));
#26339=DIRECTION('',(0.,-1.,0.));
#26340=DIRECTION('center_axis',(-1.,0.,0.));
#26341=DIRECTION('ref_axis',(0.,0.,1.));
#26342=DIRECTION('center_axis',(0.,0.923879532511284,-0.382683432365097));
#26343=DIRECTION('ref_axis',(0.,0.382683432365097,0.923879532511284));
#26344=DIRECTION('',(1.,0.,0.));
#26345=DIRECTION('',(0.678598344545853,-0.281084637714818,-0.678598344545842));
#26346=DIRECTION('',(0.678598344545855,0.281084637714819,0.67859834454584));
#26347=DIRECTION('center_axis',(0.382683432365084,0.923879532511289,0.));
#26348=DIRECTION('ref_axis',(0.,0.,1.));
#26349=DIRECTION('',(0.,0.,1.));
#26350=DIRECTION('',(0.923879532511284,-0.382683432365097,0.));
#26351=DIRECTION('center_axis',(0.,-1.,0.));
#26352=DIRECTION('ref_axis',(0.707106781186547,0.,0.707106781186547));
#26353=DIRECTION('',(0.,-0.382683432365037,0.923879532511308));
#26354=DIRECTION('center_axis',(0.,-1.,0.));
#26355=DIRECTION('ref_axis',(0.707106781186548,0.,0.707106781186548));
#26356=DIRECTION('center_axis',(0.,0.923879532511289,0.382683432365085));
#26357=DIRECTION('ref_axis',(0.,-0.382683432365085,0.923879532511289));
#26358=DIRECTION('',(0.,-0.382683432365106,0.92387953251128));
#26359=DIRECTION('',(1.,0.,0.));
#26360=DIRECTION('',(-1.,0.,0.));
#26361=DIRECTION('center_axis',(0.,-1.,0.));
#26362=DIRECTION('ref_axis',(-0.707106781186549,0.,0.707106781186546));
#26363=DIRECTION('',(-0.923879532511289,-0.382683432365085,0.));
#26364=DIRECTION('center_axis',(5.80212178386225E-16,1.,5.80212178386227E-16));
#26365=DIRECTION('ref_axis',(-0.707106781186549,0.,0.707106781186546));
#26366=DIRECTION('center_axis',(0.,-1.,0.));
#26367=DIRECTION('ref_axis',(-0.70710678118655,0.,0.707106781186545));
#26368=DIRECTION('center_axis',(-0.382683432365084,0.923879532511289,0.));
#26369=DIRECTION('ref_axis',(0.,0.,1.));
#26370=DIRECTION('',(0.,0.,1.));
#26371=DIRECTION('',(0.,0.,-1.));
#26372=DIRECTION('center_axis',(0.,-1.,0.));
#26373=DIRECTION('ref_axis',(-0.70710678118655,0.,0.707106781186545));
#26374=DIRECTION('',(0.,0.70710678118654,-0.707106781186555));
#26375=DIRECTION('',(0.707106781186548,0.707106781186548,0.));
#26376=DIRECTION('center_axis',(-0.707106781186548,0.707106781186548,0.));
#26377=DIRECTION('ref_axis',(0.,0.,1.));
#26378=DIRECTION('center_axis',(0.,1.,0.));
#26379=DIRECTION('ref_axis',(0.,0.,1.));
#26380=DIRECTION('center_axis',(0.,1.,0.));
#26381=DIRECTION('ref_axis',(1.,0.,0.));
#26382=DIRECTION('center_axis',(0.,1.,0.));
#26383=DIRECTION('ref_axis',(1.,0.,0.));
#26384=DIRECTION('center_axis',(0.,-1.,0.));
#26385=DIRECTION('ref_axis',(-1.,0.,0.));
#26386=DIRECTION('center_axis',(0.,-1.,0.));
#26387=DIRECTION('ref_axis',(-1.,0.,0.));
#26388=DIRECTION('center_axis',(0.,-1.,0.));
#26389=DIRECTION('ref_axis',(-1.,0.,0.));
#26390=DIRECTION('center_axis',(0.,-1.,0.));
#26391=DIRECTION('ref_axis',(-1.,0.,0.));
#26392=DIRECTION('center_axis',(0.,-1.,0.));
#26393=DIRECTION('ref_axis',(-1.,0.,0.));
#26394=DIRECTION('center_axis',(0.,-1.,0.));
#26395=DIRECTION('ref_axis',(-1.,0.,0.));
#26396=DIRECTION('center_axis',(0.,1.,0.));
#26397=DIRECTION('ref_axis',(1.,0.,0.));
#26398=DIRECTION('center_axis',(0.,1.,0.));
#26399=DIRECTION('ref_axis',(1.,0.,0.));
#26400=DIRECTION('center_axis',(0.,-1.,0.));
#26401=DIRECTION('ref_axis',(-1.,0.,0.));
#26402=DIRECTION('',(-0.707106781186545,0.70710678118655,-8.6595605623549E-17));
#26403=DIRECTION('center_axis',(0.,1.,0.));
#26404=DIRECTION('ref_axis',(-1.,0.,0.));
#26405=DIRECTION('center_axis',(0.,1.,0.));
#26406=DIRECTION('ref_axis',(-1.,0.,0.));
#26407=DIRECTION('',(0.,1.,0.));
#26408=DIRECTION('center_axis',(0.,-1.,0.));
#26409=DIRECTION('ref_axis',(-1.,0.,0.));
#26410=DIRECTION('center_axis',(0.,1.,0.));
#26411=DIRECTION('ref_axis',(1.,0.,0.));
#26412=DIRECTION('',(0.707106781186548,-0.707106781186548,-8.65956056235493E-17));
#26413=DIRECTION('center_axis',(0.,-1.,0.));
#26414=DIRECTION('ref_axis',(1.,0.,0.));
#26415=DIRECTION('center_axis',(0.,-1.,0.));
#26416=DIRECTION('ref_axis',(1.,0.,0.));
#26417=DIRECTION('center_axis',(0.,1.,0.));
#26418=DIRECTION('ref_axis',(-1.,0.,0.));
#26419=DIRECTION('center_axis',(0.,1.,0.));
#26420=DIRECTION('ref_axis',(1.,0.,0.));
#26421=DIRECTION('',(0.,1.,0.));
#26422=DIRECTION('center_axis',(0.,1.,0.));
#26423=DIRECTION('ref_axis',(-1.,0.,0.));
#26424=DIRECTION('',(0.707106781186545,0.70710678118655,8.6595605623549E-17));
#26425=DIRECTION('center_axis',(0.,1.,0.));
#26426=DIRECTION('ref_axis',(-1.,0.,0.));
#26427=DIRECTION('center_axis',(0.,-1.,0.));
#26428=DIRECTION('ref_axis',(0.,0.,-1.));
#26429=DIRECTION('center_axis',(0.,1.,0.));
#26430=DIRECTION('ref_axis',(1.,0.,0.));
#26431=DIRECTION('',(0.707106781186548,-0.707106781186548,-8.65956056235493E-17));
#26432=DIRECTION('center_axis',(0.,-1.,0.));
#26433=DIRECTION('ref_axis',(1.,0.,0.));
#26434=DIRECTION('center_axis',(0.,-1.,0.));
#26435=DIRECTION('ref_axis',(1.,0.,0.));
#26436=DIRECTION('center_axis',(0.,1.,0.));
#26437=DIRECTION('ref_axis',(-1.,0.,0.));
#26438=DIRECTION('center_axis',(0.,1.,0.));
#26439=DIRECTION('ref_axis',(-1.,0.,0.));
#26440=DIRECTION('',(0.,1.,0.));
#26441=DIRECTION('center_axis',(0.,-1.,0.));
#26442=DIRECTION('ref_axis',(-1.,0.,0.));
#26443=DIRECTION('',(-0.707106781186545,0.70710678118655,-8.6595605623549E-17));
#26444=DIRECTION('center_axis',(0.,1.,0.));
#26445=DIRECTION('ref_axis',(1.,0.,0.));
#26446=DIRECTION('',(0.707106781186553,-0.707106781186542,-8.659560562355E-17));
#26447=DIRECTION('center_axis',(0.,-1.,0.));
#26448=DIRECTION('ref_axis',(1.,0.,0.));
#26449=DIRECTION('center_axis',(0.,-1.,0.));
#26450=DIRECTION('ref_axis',(1.,0.,0.));
#26451=DIRECTION('center_axis',(0.,1.,0.));
#26452=DIRECTION('ref_axis',(-1.,0.,0.));
#26453=DIRECTION('center_axis',(0.,1.,0.));
#26454=DIRECTION('ref_axis',(-1.,0.,0.));
#26455=DIRECTION('',(0.,1.,0.));
#26456=DIRECTION('center_axis',(0.,-1.,0.));
#26457=DIRECTION('ref_axis',(-1.,0.,0.));
#26458=DIRECTION('',(-0.70710678118655,0.707106781186545,-8.65956056235496E-17));
#26459=DIRECTION('center_axis',(0.,1.,0.));
#26460=DIRECTION('ref_axis',(1.,0.,0.));
#26461=DIRECTION('',(0.707106781186548,-0.707106781186548,-8.65956056235493E-17));
#26462=DIRECTION('center_axis',(0.,-1.,0.));
#26463=DIRECTION('ref_axis',(1.,0.,0.));
#26464=DIRECTION('center_axis',(0.,-1.,0.));
#26465=DIRECTION('ref_axis',(1.,0.,0.));
#26466=DIRECTION('center_axis',(0.,1.,0.));
#26467=DIRECTION('ref_axis',(-1.,0.,0.));
#26468=DIRECTION('center_axis',(0.,1.,0.));
#26469=DIRECTION('ref_axis',(-1.,0.,0.));
#26470=DIRECTION('',(0.,1.,0.));
#26471=DIRECTION('center_axis',(0.,-1.,0.));
#26472=DIRECTION('ref_axis',(-1.,0.,0.));
#26473=DIRECTION('',(-0.707106781186545,0.70710678118655,-8.6595605623549E-17));
#26474=DIRECTION('center_axis',(0.,-1.,0.));
#26475=DIRECTION('ref_axis',(-1.,0.,0.));
#26476=DIRECTION('',(-0.70710678118655,0.707106781186545,-8.65956056235497E-17));
#26477=DIRECTION('center_axis',(0.,1.,0.));
#26478=DIRECTION('ref_axis',(-1.,0.,0.));
#26479=DIRECTION('center_axis',(0.,1.,0.));
#26480=DIRECTION('ref_axis',(-1.,0.,0.));
#26481=DIRECTION('',(0.,1.,0.));
#26482=DIRECTION('center_axis',(0.,1.,0.));
#26483=DIRECTION('ref_axis',(1.,0.,0.));
#26484=DIRECTION('center_axis',(0.,-1.,0.));
#26485=DIRECTION('ref_axis',(-1.,0.,0.));
#26486=DIRECTION('',(-0.70710678118655,0.707106781186545,-8.65956056235496E-17));
#26487=DIRECTION('center_axis',(0.,1.,0.));
#26488=DIRECTION('ref_axis',(-1.,0.,0.));
#26489=DIRECTION('center_axis',(0.,1.,0.));
#26490=DIRECTION('ref_axis',(-1.,0.,0.));
#26491=DIRECTION('',(0.,1.,0.));
#26492=DIRECTION('center_axis',(0.,1.,0.));
#26493=DIRECTION('ref_axis',(1.,0.,0.));
#26494=DIRECTION('center_axis',(0.,-1.,0.));
#26495=DIRECTION('ref_axis',(-1.,0.,0.));
#26496=DIRECTION('',(-0.707106781186547,0.707106781186548,-8.65956056235492E-17));
#26497=DIRECTION('center_axis',(0.,1.,0.));
#26498=DIRECTION('ref_axis',(-1.,0.,0.));
#26499=DIRECTION('center_axis',(0.,1.,0.));
#26500=DIRECTION('ref_axis',(-1.,0.,0.));
#26501=DIRECTION('',(0.,1.,0.));
#26502=DIRECTION('center_axis',(0.,1.,0.));
#26503=DIRECTION('ref_axis',(1.,0.,0.));
#26504=DIRECTION('center_axis',(0.,0.,1.));
#26505=DIRECTION('ref_axis',(1.,0.,0.));
#26506=DIRECTION('center_axis',(0.,0.,1.));
#26507=DIRECTION('ref_axis',(1.,0.,0.));
#26508=DIRECTION('',(0.923879532511284,1.1314261122877E-16,-0.382683432365096));
#26509=DIRECTION('center_axis',(0.,0.,-1.));
#26510=DIRECTION('ref_axis',(1.,0.,0.));
#26511=DIRECTION('center_axis',(0.,0.,1.));
#26512=DIRECTION('ref_axis',(1.,0.,0.));
#26513=DIRECTION('center_axis',(0.,0.,1.));
#26514=DIRECTION('ref_axis',(-1.,0.,0.));
#26515=DIRECTION('center_axis',(0.,0.,1.));
#26516=DIRECTION('ref_axis',(-1.,0.,0.));
#26517=DIRECTION('',(-0.707106781186543,-8.65956056235488E-17,0.707106781186552));
#26518=DIRECTION('center_axis',(0.,0.,1.));
#26519=DIRECTION('ref_axis',(1.,0.,0.));
#26520=DIRECTION('',(0.,-1.,0.));
#26521=DIRECTION('center_axis',(0.,0.,1.));
#26522=DIRECTION('ref_axis',(-1.,0.,0.));
#26523=DIRECTION('center_axis',(0.,0.,-1.));
#26524=DIRECTION('ref_axis',(-1.,0.,0.));
#26525=DIRECTION('center_axis',(0.,0.,-1.));
#26526=DIRECTION('ref_axis',(-1.,0.,0.));
#26527=DIRECTION('',(0.382683432365085,-4.68652040532624E-17,0.923879532511289));
#26528=DIRECTION('center_axis',(0.,0.,1.));
#26529=DIRECTION('ref_axis',(1.,0.,0.));
#26530=DIRECTION('center_axis',(0.,0.,1.));
#26531=DIRECTION('ref_axis',(1.,0.,0.));
#26532=DIRECTION('',(0.,0.,1.));
#26533=DIRECTION('center_axis',(0.,0.,1.));
#26534=DIRECTION('ref_axis',(1.,0.,0.));
#26535=DIRECTION('',(-0.857167300702113,-1.04972719113862E-16,0.515038074910052));
#26536=DIRECTION('center_axis',(0.,0.,-1.));
#26537=DIRECTION('ref_axis',(-1.,0.,0.));
#26538=DIRECTION('',(0.857167300702112,-1.04972719113862E-16,-0.515038074910054));
#26539=DIRECTION('center_axis',(0.,0.,-1.));
#26540=DIRECTION('ref_axis',(1.,0.,0.));
#26541=DIRECTION('center_axis',(0.,0.,-1.));
#26542=DIRECTION('ref_axis',(-1.,0.,0.));
#26543=DIRECTION('',(0.,0.,-1.));
#26544=DIRECTION('center_axis',(0.,0.,-1.));
#26545=DIRECTION('ref_axis',(1.,0.,0.));
#26546=DIRECTION('center_axis',(0.,0.,-1.));
#26547=DIRECTION('ref_axis',(-1.,0.,0.));
#26548=DIRECTION('',(0.707106781186546,-8.65956056235491E-17,-0.707106781186549));
#26549=DIRECTION('center_axis',(0.,0.,-1.));
#26550=DIRECTION('ref_axis',(-1.,0.,0.));
#26551=DIRECTION('',(0.857167300702112,-1.04972719113862E-16,-0.515038074910054));
#26552=DIRECTION('center_axis',(0.,0.,-1.));
#26553=DIRECTION('ref_axis',(1.,0.,0.));
#26554=DIRECTION('center_axis',(0.,0.,-1.));
#26555=DIRECTION('ref_axis',(-1.,0.,0.));
#26556=DIRECTION('',(0.,0.,-1.));
#26557=DIRECTION('center_axis',(0.,0.,-1.));
#26558=DIRECTION('ref_axis',(1.,0.,0.));
#26559=DIRECTION('center_axis',(0.,0.,-1.));
#26560=DIRECTION('ref_axis',(-1.,0.,0.));
#26561=DIRECTION('',(0.707106781186547,-8.65956056235493E-17,-0.707106781186548));
#26562=DIRECTION('center_axis',(0.,0.,-1.));
#26563=DIRECTION('ref_axis',(-1.,0.,0.));
#26564=DIRECTION('',(0.857167300702112,-1.04972719113862E-16,-0.515038074910054));
#26565=DIRECTION('center_axis',(0.,0.,-1.));
#26566=DIRECTION('ref_axis',(1.,0.,0.));
#26567=DIRECTION('center_axis',(0.,0.,-1.));
#26568=DIRECTION('ref_axis',(-1.,0.,0.));
#26569=DIRECTION('',(0.,0.,-1.));
#26570=DIRECTION('center_axis',(0.,0.,-1.));
#26571=DIRECTION('ref_axis',(1.,0.,0.));
#26572=DIRECTION('center_axis',(0.,0.,-1.));
#26573=DIRECTION('ref_axis',(-1.,0.,0.));
#26574=DIRECTION('',(0.707106781186546,-8.65956056235491E-17,-0.707106781186549));
#26575=DIRECTION('center_axis',(0.,1.,0.));
#26576=DIRECTION('ref_axis',(-1.,0.,0.));
#26577=DIRECTION('',(0.52999894000318,0.847998304005088,-6.49061505426384E-17));
#26578=DIRECTION('center_axis',(0.,1.,0.));
#26579=DIRECTION('ref_axis',(-1.,0.,0.));
#26580=DIRECTION('',(0.529998940003178,0.847998304005089,-6.49061505426383E-17));
#26581=DIRECTION('center_axis',(0.,1.,0.));
#26582=DIRECTION('ref_axis',(-1.,0.,0.));
#26583=DIRECTION('',(0.529998940003178,0.847998304005089,-6.49061505426382E-17));
#26584=DIRECTION('center_axis',(0.,1.,0.));
#26585=DIRECTION('ref_axis',(-1.,0.,0.));
#26586=DIRECTION('',(0.857167300702112,0.515038074910054,-1.04972719113862E-16));
#26587=DIRECTION('center_axis',(0.,1.,0.));
#26588=DIRECTION('ref_axis',(1.,0.,0.));
#26589=DIRECTION('center_axis',(0.,1.,0.));
#26590=DIRECTION('ref_axis',(-1.,0.,0.));
#26591=DIRECTION('',(0.,1.,0.));
#26592=DIRECTION('center_axis',(0.,1.,0.));
#26593=DIRECTION('ref_axis',(1.,0.,0.));
#26594=DIRECTION('center_axis',(0.,1.,0.));
#26595=DIRECTION('ref_axis',(-1.,0.,0.));
#26596=DIRECTION('',(0.707106781186548,0.707106781186547,-8.65956056235493E-17));
#26597=DIRECTION('center_axis',(0.,1.,0.));
#26598=DIRECTION('ref_axis',(-1.,0.,0.));
#26599=DIRECTION('',(0.857167300702112,0.515038074910054,-1.04972719113862E-16));
#26600=DIRECTION('center_axis',(0.,1.,0.));
#26601=DIRECTION('ref_axis',(1.,0.,0.));
#26602=DIRECTION('center_axis',(0.,1.,0.));
#26603=DIRECTION('ref_axis',(-1.,0.,0.));
#26604=DIRECTION('',(0.,1.,0.));
#26605=DIRECTION('center_axis',(0.,1.,0.));
#26606=DIRECTION('ref_axis',(1.,0.,0.));
#26607=DIRECTION('center_axis',(0.,1.,0.));
#26608=DIRECTION('ref_axis',(-1.,0.,0.));
#26609=DIRECTION('',(0.707106781186548,0.707106781186547,-8.65956056235493E-17));
#26610=DIRECTION('center_axis',(0.,1.,0.));
#26611=DIRECTION('ref_axis',(-1.,0.,0.));
#26612=DIRECTION('',(0.857167300702112,0.515038074910054,-1.04972719113862E-16));
#26613=DIRECTION('center_axis',(0.,1.,0.));
#26614=DIRECTION('ref_axis',(1.,0.,0.));
#26615=DIRECTION('center_axis',(0.,1.,0.));
#26616=DIRECTION('ref_axis',(-1.,0.,0.));
#26617=DIRECTION('',(0.,1.,0.));
#26618=DIRECTION('center_axis',(0.,1.,0.));
#26619=DIRECTION('ref_axis',(1.,0.,0.));
#26620=DIRECTION('center_axis',(0.,1.,0.));
#26621=DIRECTION('ref_axis',(-1.,0.,0.));
#26622=DIRECTION('',(0.707106781186546,0.707106781186549,-8.65956056235491E-17));
#26623=DIRECTION('center_axis',(0.,0.70710678118654,0.707106781186555));
#26624=DIRECTION('ref_axis',(1.,0.,0.));
#26625=DIRECTION('center_axis',(0.,1.,0.));
#26626=DIRECTION('ref_axis',(0.707106781186547,0.,0.707106781186547));
#32248=CARTESIAN_POINT('',(0.,0.,0.));
#32249=CARTESIAN_POINT('Origin',(1.55,1.4106066017178,1.2843933982822));
#32250=CARTESIAN_POINT('',(6.09,1.4,1.31));
#32251=CARTESIAN_POINT('',(-6.09,1.4,1.31));
#32252=CARTESIAN_POINT('',(1.55,1.4,1.31));
#32253=CARTESIAN_POINT('',(-6.1412132034356,1.4212132034356,1.2587867965644));
#32254=CARTESIAN_POINT('',(-6.09,1.4,1.31));
#32255=CARTESIAN_POINT('',(6.1412132034356,1.4212132034356,1.2587867965644));
#32256=CARTESIAN_POINT('',(1.55,1.4212132034356,1.2587867965644));
#32257=CARTESIAN_POINT('',(6.1412132034356,1.4212132034356,1.2587867965644));
#32258=CARTESIAN_POINT('Origin',(-6.1156066017178,1.4106066017178,6.825));
#32259=CARTESIAN_POINT('',(-6.09,1.4,15.6));
#32260=CARTESIAN_POINT('',(-6.09,1.4,6.825));
#32261=CARTESIAN_POINT('',(-6.1412132034356,1.4212132034356,15.6));
#32262=CARTESIAN_POINT('',(-6.09,1.4,15.6));
#32263=CARTESIAN_POINT('',(-6.1412132034356,1.4212132034356,6.825));
#32264=CARTESIAN_POINT('Origin',(-5.6,1.4106066017178,15.6));
#32265=CARTESIAN_POINT('',(-5.6,1.4,16.09));
#32266=CARTESIAN_POINT('',(-5.6,1.4212132034356,16.1412132034356));
#32267=CARTESIAN_POINT('',(-5.6,1.4,16.09));
#32268=CARTESIAN_POINT('Origin',(-5.6,1.4212132034356,15.6));
#32269=CARTESIAN_POINT('Origin',(-5.6,1.4,15.6));
#32270=CARTESIAN_POINT('Origin',(-1.55,1.4106066017178,16.1156066017178));
#32271=CARTESIAN_POINT('',(5.6,1.4,16.09));
#32272=CARTESIAN_POINT('',(5.6,1.4212132034356,16.1412132034356));
#32273=CARTESIAN_POINT('',(5.6,1.4,16.09));
#32274=CARTESIAN_POINT('',(-1.55,1.4212132034356,16.1412132034356));
#32275=CARTESIAN_POINT('',(-1.55,1.4,16.09));
#32276=CARTESIAN_POINT('Origin',(5.6,1.4106066017178,15.6));
#32277=CARTESIAN_POINT('',(6.09,1.4,15.6));
#32278=CARTESIAN_POINT('',(6.1412132034356,1.42121320343559,15.6));
#32279=CARTESIAN_POINT('',(6.09,1.4,15.6));
#32280=CARTESIAN_POINT('Origin',(5.6,1.4212132034356,15.6));
#32281=CARTESIAN_POINT('Origin',(5.6,1.4,15.6));
#32282=CARTESIAN_POINT('Origin',(6.1156066017178,1.4106066017178,10.575));
#32283=CARTESIAN_POINT('',(6.1412132034356,1.4212132034356,10.575));
#32284=CARTESIAN_POINT('',(6.09,1.4,10.575));
#32285=CARTESIAN_POINT('Origin',(5.6,1.44,15.6));
#32286=CARTESIAN_POINT('',(6.1787867965644,1.4587867965644,15.6));
#32287=CARTESIAN_POINT('',(6.2,1.48,15.6));
#32288=CARTESIAN_POINT('',(5.6,1.4587867965644,16.1787867965644));
#32289=CARTESIAN_POINT('Origin',(5.6,1.4587867965644,15.6));
#32290=CARTESIAN_POINT('',(5.6,1.48,16.2));
#32291=CARTESIAN_POINT('Origin',(6.16,1.44,12.45));
#32292=CARTESIAN_POINT('',(6.1787867965644,1.4587867965644,1.2212132034356));
#32293=CARTESIAN_POINT('',(6.12,1.4,1.28));
#32294=CARTESIAN_POINT('',(6.1787867965644,1.4587867965644,14.325));
#32295=CARTESIAN_POINT('Origin',(3.1,1.44,1.24));
#32296=CARTESIAN_POINT('',(-6.1787867965644,1.4587867965644,1.2212132034356));
#32297=CARTESIAN_POINT('',(-6.12,1.4,1.28));
#32298=CARTESIAN_POINT('',(4.65,1.4587867965644,1.2212132034356));
#32299=CARTESIAN_POINT('Origin',(0.,1.4,8.7));
#32300=CARTESIAN_POINT('',(3.33,1.4,8.5));
#32301=CARTESIAN_POINT('Origin',(0.,1.4,8.5));
#32302=CARTESIAN_POINT('',(-4.2,1.4,8.5));
#32303=CARTESIAN_POINT('Origin',(-4.4,1.4,8.5));
#32304=CARTESIAN_POINT('',(5.06823591024675,1.4,11.175));
#32305=CARTESIAN_POINT('Origin',(4.63323591024675,1.4,11.175));
#32306=CARTESIAN_POINT('',(0.434999999999999,1.4,3.15));
#32307=CARTESIAN_POINT('Origin',(-9.82779056315751E-16,1.4,3.15));
#32308=CARTESIAN_POINT('',(-4.19823591024675,1.4,11.175));
#32309=CARTESIAN_POINT('Origin',(-4.63323591024675,1.4,11.175));
#32310=CARTESIAN_POINT('',(2.4,1.4,4.68948822334847));
#32311=CARTESIAN_POINT('Origin',(2.2,1.4,4.68948822334847));
#32312=CARTESIAN_POINT('',(2.4,1.4,12.3105117766515));
#32313=CARTESIAN_POINT('Origin',(2.2,1.4,12.3105117766515));
#32314=CARTESIAN_POINT('Origin',(4.65,1.4843933982822,1.2106066017178));
#32315=CARTESIAN_POINT('',(6.185,1.4737867965644,1.215));
#32316=CARTESIAN_POINT('',(5.25345910630655,-0.775151862895448,2.14654089369344));
#32317=CARTESIAN_POINT('',(-6.185,1.4737867965644,1.215));
#32318=CARTESIAN_POINT('',(-5.3780051976814,-0.474470999957732,2.02199480231859));
#32319=CARTESIAN_POINT('',(-6.17,1.51,1.2));
#32320=CARTESIAN_POINT('',(-5.50243230506491,3.12165098291439,0.532432305064926));
#32321=CARTESIAN_POINT('',(6.17,1.51,1.2));
#32322=CARTESIAN_POINT('',(4.65,1.51,1.2));
#32323=CARTESIAN_POINT('',(6.09642135623731,1.6876345596729,1.12642135623731));
#32324=CARTESIAN_POINT('Origin',(6.2,1.4,1.2));
#32325=CARTESIAN_POINT('',(-6.17,3.09,1.2));
#32326=CARTESIAN_POINT('',(-6.17,1.4,1.2));
#32327=CARTESIAN_POINT('',(6.17,3.09,1.2));
#32328=CARTESIAN_POINT('',(4.65,3.09,1.2));
#32329=CARTESIAN_POINT('',(6.17,1.4,1.2));
#32330=CARTESIAN_POINT('',(-4.195,2.3,1.2));
#32331=CARTESIAN_POINT('Origin',(-4.5,2.3,1.2));
#32332=CARTESIAN_POINT('',(0.305,2.3,1.2));
#32333=CARTESIAN_POINT('Origin',(0.,2.3,1.2));
#32334=CARTESIAN_POINT('',(4.805,2.3,1.2));
#32335=CARTESIAN_POINT('Origin',(4.5,2.3,1.2));
#32336=CARTESIAN_POINT('Origin',(-6.185,1.4,1.215));
#32337=CARTESIAN_POINT('',(-6.2,1.51,1.23));
#32338=CARTESIAN_POINT('',(-6.2943363256585,1.73774803682919,1.3243363256585));
#32339=CARTESIAN_POINT('',(-6.2,3.09,1.23));
#32340=CARTESIAN_POINT('',(-6.2,1.4,1.23));
#32341=CARTESIAN_POINT('',(-6.185,3.1262132034356,1.215));
#32342=CARTESIAN_POINT('',(-6.57188789144717,2.19218320878592,1.60188789144716));
#32343=CARTESIAN_POINT('',(-5.22488073927622,0.808280262700718,0.254880739276242));
#32344=CARTESIAN_POINT('Origin',(-6.1893933982822,1.4843933982822,3.075));
#32345=CARTESIAN_POINT('',(-6.1787867965644,1.4587867965644,15.6));
#32346=CARTESIAN_POINT('',(-6.1787867965644,1.4587867965644,3.075));
#32347=CARTESIAN_POINT('',(-6.2,1.51,15.6));
#32348=CARTESIAN_POINT('',(-6.2,1.51,15.6));
#32349=CARTESIAN_POINT('',(-6.2,1.51,3.075));
#32350=CARTESIAN_POINT('Origin',(6.1893933982822,1.4843933982822,14.325));
#32351=CARTESIAN_POINT('',(6.2,1.51,1.23));
#32352=CARTESIAN_POINT('',(7.01287146820574,3.47244532300839,2.04287146820574));
#32353=CARTESIAN_POINT('',(6.2,1.51,15.6));
#32354=CARTESIAN_POINT('',(6.2,1.51,14.325));
#32355=CARTESIAN_POINT('',(6.2,1.51,15.6));
#32356=CARTESIAN_POINT('Origin',(5.6,1.4843933982822,15.6));
#32357=CARTESIAN_POINT('',(5.6,1.51,16.2));
#32358=CARTESIAN_POINT('',(5.6,1.51,16.2));
#32359=CARTESIAN_POINT('Origin',(5.6,1.51,15.6));
#32360=CARTESIAN_POINT('Origin',(-4.65,1.4843933982822,16.1893933982822));
#32361=CARTESIAN_POINT('',(-5.6,1.51,16.2));
#32362=CARTESIAN_POINT('',(-5.6,1.4587867965644,16.1787867965644));
#32363=CARTESIAN_POINT('',(-5.6,1.51,16.2));
#32364=CARTESIAN_POINT('',(-4.65,1.4587867965644,16.1787867965644));
#32365=CARTESIAN_POINT('',(-4.65,1.51,16.2));
#32366=CARTESIAN_POINT('Origin',(-5.6,1.4843933982822,15.6));
#32367=CARTESIAN_POINT('Origin',(-5.6,1.4587867965644,15.6));
#32368=CARTESIAN_POINT('Origin',(-5.6,1.51,15.6));
#32369=CARTESIAN_POINT('Origin',(-3.1,1.44,16.16));
#32370=CARTESIAN_POINT('',(-5.6,1.48,16.2));
#32371=CARTESIAN_POINT('Origin',(-5.6,1.44,15.6));
#32372=CARTESIAN_POINT('',(-6.2,1.48,15.6));
#32373=CARTESIAN_POINT('Origin',(-6.16,1.44,4.95));
#32374=CARTESIAN_POINT('Origin',(4.65,3.1156066017178,1.2106066017178));
#32375=CARTESIAN_POINT('',(-6.1787867965644,3.1412132034356,1.2212132034356));
#32376=CARTESIAN_POINT('',(-6.2,3.09,1.2));
#32377=CARTESIAN_POINT('',(6.1787867965644,3.1412132034356,1.2212132034356));
#32378=CARTESIAN_POINT('',(4.65,3.1412132034356,1.2212132034356));
#32379=CARTESIAN_POINT('',(6.185,3.1262132034356,1.215));
#32380=CARTESIAN_POINT('',(6.1787867965644,3.1412132034356,1.2212132034356));
#32381=CARTESIAN_POINT('',(5.81886979044864,2.24229668594221,0.848869790448636));
#32382=CARTESIAN_POINT('Origin',(6.185,1.4,1.215));
#32383=CARTESIAN_POINT('',(6.2,3.09,1.23));
#32384=CARTESIAN_POINT('',(7.29042303399442,0.457485922606718,2.32042303399443));
#32385=CARTESIAN_POINT('',(6.2,1.4,1.23));
#32386=CARTESIAN_POINT('Origin',(6.2,1.4,16.2));
#32387=CARTESIAN_POINT('',(6.2,3.09,15.6));
#32388=CARTESIAN_POINT('',(6.2,3.09,14.325));
#32389=CARTESIAN_POINT('',(6.2,1.4,15.6));
#32390=CARTESIAN_POINT('Origin',(6.1893933982822,3.1156066017178,14.325));
#32391=CARTESIAN_POINT('',(6.1787867965644,3.1412132034356,15.6));
#32392=CARTESIAN_POINT('',(6.1787867965644,3.1412132034356,14.325));
#32393=CARTESIAN_POINT('',(6.2,3.09,15.6));
#32394=CARTESIAN_POINT('Origin',(-6.1893933982822,3.1156066017178,3.075));
#32395=CARTESIAN_POINT('',(-6.2,3.09,15.6));
#32396=CARTESIAN_POINT('',(-6.2,3.09,3.075));
#32397=CARTESIAN_POINT('',(-6.1787867965644,3.1412132034356,15.6));
#32398=CARTESIAN_POINT('',(-6.2,3.09,15.6));
#32399=CARTESIAN_POINT('',(-6.1787867965644,3.1412132034356,3.075));
#32400=CARTESIAN_POINT('Origin',(-5.6,3.1156066017178,15.6));
#32401=CARTESIAN_POINT('',(-5.6,3.09,16.2));
#32402=CARTESIAN_POINT('',(-5.6,3.1412132034356,16.1787867965644));
#32403=CARTESIAN_POINT('',(-5.6,3.09,16.2));
#32404=CARTESIAN_POINT('Origin',(-5.6,3.1412132034356,15.6));
#32405=CARTESIAN_POINT('Origin',(-5.6,3.09,15.6));
#32406=CARTESIAN_POINT('Origin',(-4.65,3.1156066017178,16.1893933982822));
#32407=CARTESIAN_POINT('',(5.6,3.09,16.2));
#32408=CARTESIAN_POINT('',(5.6,3.1412132034356,16.1787867965644));
#32409=CARTESIAN_POINT('',(5.6,3.09,16.2));
#32410=CARTESIAN_POINT('',(-4.65,3.1412132034356,16.1787867965644));
#32411=CARTESIAN_POINT('',(-4.65,3.09,16.2));
#32412=CARTESIAN_POINT('Origin',(5.6,3.1156066017178,15.6));
#32413=CARTESIAN_POINT('Origin',(5.6,3.1412132034356,15.6));
#32414=CARTESIAN_POINT('Origin',(5.6,3.09,15.6));
#32415=CARTESIAN_POINT('Origin',(5.6,3.16,15.6));
#32416=CARTESIAN_POINT('',(6.1412132034356,3.1787867965644,15.6));
#32417=CARTESIAN_POINT('',(6.2,3.12,15.6));
#32418=CARTESIAN_POINT('',(5.6,3.17878679656441,16.1412132034356));
#32419=CARTESIAN_POINT('Origin',(5.6,3.1787867965644,15.6));
#32420=CARTESIAN_POINT('',(5.6,3.12,16.2));
#32421=CARTESIAN_POINT('Origin',(6.16,3.16,12.45));
#32422=CARTESIAN_POINT('',(6.1412132034356,3.1787867965644,1.2587867965644));
#32423=CARTESIAN_POINT('',(6.12,3.2,1.28));
#32424=CARTESIAN_POINT('',(6.1412132034356,3.1787867965644,10.575));
#32425=CARTESIAN_POINT('Origin',(3.1,3.16,1.24));
#32426=CARTESIAN_POINT('',(-6.1412132034356,3.1787867965644,1.2587867965644));
#32427=CARTESIAN_POINT('',(-6.12,3.2,1.28));
#32428=CARTESIAN_POINT('',(1.55,3.1787867965644,1.2587867965644));
#32429=CARTESIAN_POINT('Origin',(-5.6,1.4,15.6));
#32430=CARTESIAN_POINT('',(-5.6,1.4,16.2));
#32431=CARTESIAN_POINT('',(-6.2,1.4,15.6));
#32432=CARTESIAN_POINT('Origin',(-6.2,1.4,1.2));
#32433=CARTESIAN_POINT('Origin',(1.55,3.1893933982822,1.2843933982822));
#32434=CARTESIAN_POINT('',(-6.09,3.2,1.31));
#32435=CARTESIAN_POINT('',(6.09,3.2,1.31));
#32436=CARTESIAN_POINT('',(1.55,3.2,1.31));
#32437=CARTESIAN_POINT('',(6.09,3.2,1.31));
#32438=CARTESIAN_POINT('',(-6.1412132034356,3.1787867965644,1.2587867965644));
#32439=CARTESIAN_POINT('Origin',(6.1156066017178,3.1893933982822,10.575));
#32440=CARTESIAN_POINT('',(6.09,3.2,15.6));
#32441=CARTESIAN_POINT('',(6.09,3.2,10.575));
#32442=CARTESIAN_POINT('',(6.09,3.2,15.6));
#32443=CARTESIAN_POINT('Origin',(5.6,3.1893933982822,15.6));
#32444=CARTESIAN_POINT('',(5.6,3.2,16.09));
#32445=CARTESIAN_POINT('',(5.6,3.2,16.09));
#32446=CARTESIAN_POINT('Origin',(5.6,3.2,15.6));
#32447=CARTESIAN_POINT('Origin',(-1.55,3.1893933982822,16.1156066017178));
#32448=CARTESIAN_POINT('',(-5.6,3.2,16.09));
#32449=CARTESIAN_POINT('',(-5.6,3.1787867965644,16.1412132034356));
#32450=CARTESIAN_POINT('',(-5.6,3.2,16.09));
#32451=CARTESIAN_POINT('',(-1.55,3.1787867965644,16.1412132034356));
#32452=CARTESIAN_POINT('',(-1.55,3.2,16.09));
#32453=CARTESIAN_POINT('Origin',(-5.6,3.1893933982822,15.6));
#32454=CARTESIAN_POINT('',(-6.09,3.2,15.6));
#32455=CARTESIAN_POINT('',(-6.1412132034356,3.1787867965644,15.6));
#32456=CARTESIAN_POINT('',(-6.09,3.2,15.6));
#32457=CARTESIAN_POINT('Origin',(-5.6,3.1787867965644,15.6));
#32458=CARTESIAN_POINT('Origin',(-5.6,3.2,15.6));
#32459=CARTESIAN_POINT('Origin',(-6.1156066017178,3.1893933982822,6.825));
#32460=CARTESIAN_POINT('',(-6.1412132034356,3.1787867965644,6.825));
#32461=CARTESIAN_POINT('',(-6.09,3.2,6.825));
#32462=CARTESIAN_POINT('Origin',(-5.6,3.16,15.6));
#32463=CARTESIAN_POINT('',(-5.6,3.12,16.2));
#32464=CARTESIAN_POINT('',(-6.2,3.12,15.6));
#32465=CARTESIAN_POINT('Origin',(-6.16,3.16,4.95));
#32466=CARTESIAN_POINT('Origin',(0.,3.2,8.7));
#32467=CARTESIAN_POINT('',(-3.805,3.2,8.5));
#32468=CARTESIAN_POINT('Origin',(0.,3.2,8.5));
#32469=CARTESIAN_POINT('',(-4.6,3.2,8.5));
#32470=CARTESIAN_POINT('Origin',(-4.4,3.2,8.5));
#32471=CARTESIAN_POINT('',(0.423749999999999,3.2,3.15));
#32472=CARTESIAN_POINT('Origin',(-9.82779056315751E-16,3.2,3.15));
#32473=CARTESIAN_POINT('',(5.05698591024675,3.2,11.175));
#32474=CARTESIAN_POINT('Origin',(4.63323591024675,3.2,11.175));
#32475=CARTESIAN_POINT('',(-1.995,3.2,4.68948822334847));
#32476=CARTESIAN_POINT('Origin',(-2.2,3.2,4.68948822334847));
#32477=CARTESIAN_POINT('',(-1.995,3.2,12.3105117766515));
#32478=CARTESIAN_POINT('Origin',(-2.2,3.2,12.3105117766515));
#32479=CARTESIAN_POINT('',(4.605,3.2,8.5));
#32480=CARTESIAN_POINT('Origin',(4.4,3.2,8.5));
#32481=CARTESIAN_POINT('',(-4.20948591024675,3.2,11.175));
#32482=CARTESIAN_POINT('Origin',(-4.63323591024675,3.2,11.175));
#32483=CARTESIAN_POINT('',(2.,3.2,4.68948822334847));
#32484=CARTESIAN_POINT('Origin',(2.2,3.2,4.68948822334847));
#32485=CARTESIAN_POINT('',(2.,3.2,12.3105117766515));
#32486=CARTESIAN_POINT('Origin',(2.2,3.2,12.3105117766515));
#32487=CARTESIAN_POINT('Origin',(0.,1.415,8.5));
#32488=CARTESIAN_POINT('',(3.3,1.43,8.5));
#32489=CARTESIAN_POINT('',(3.315,1.415,8.5));
#32490=CARTESIAN_POINT('Origin',(0.,1.43,8.5));
#32491=CARTESIAN_POINT('Origin',(0.,2.3,8.5));
#32492=CARTESIAN_POINT('',(3.3,1.87,8.5));
#32493=CARTESIAN_POINT('',(3.3,2.3,8.5));
#32494=CARTESIAN_POINT('Origin',(0.,1.87,8.5));
#32495=CARTESIAN_POINT('Origin',(0.,3.185,8.5));
#32496=CARTESIAN_POINT('',(-3.775,3.17,8.5));
#32497=CARTESIAN_POINT('',(-3.79,3.185,8.5));
#32498=CARTESIAN_POINT('',(3.775,3.17,8.5));
#32499=CARTESIAN_POINT('Origin',(0.,3.17,8.5));
#32500=CARTESIAN_POINT('Origin',(0.,3.17,8.5));
#32501=CARTESIAN_POINT('Origin',(0.,2.55,8.5));
#32502=CARTESIAN_POINT('',(3.775,1.9,8.5));
#32503=CARTESIAN_POINT('Origin',(0.,1.9,8.5));
#32504=CARTESIAN_POINT('',(3.775,2.55,8.5));
#32505=CARTESIAN_POINT('Origin',(0.,1.885,8.5));
#32506=CARTESIAN_POINT('',(3.33,1.9,8.5));
#32507=CARTESIAN_POINT('',(3.315,1.885,8.5));
#32508=CARTESIAN_POINT('Origin',(0.,1.9,8.5));
#32509=CARTESIAN_POINT('Origin',(-3.775,1.9,8.5));
#32510=CARTESIAN_POINT('Origin',(2.2,3.185,12.3105117766515));
#32511=CARTESIAN_POINT('',(2.03,3.17,12.3105117766515));
#32512=CARTESIAN_POINT('',(2.015,3.185,12.3105117766515));
#32513=CARTESIAN_POINT('',(2.37,3.17,12.3105117766515));
#32514=CARTESIAN_POINT('Origin',(2.2,3.17,12.3105117766515));
#32515=CARTESIAN_POINT('Origin',(2.2,3.17,12.3105117766515));
#32516=CARTESIAN_POINT('Origin',(2.2,2.275,12.3105117766515));
#32517=CARTESIAN_POINT('',(2.37,1.43,12.3105117766515));
#32518=CARTESIAN_POINT('Origin',(2.2,1.43,12.3105117766515));
#32519=CARTESIAN_POINT('',(2.37,2.275,12.3105117766515));
#32520=CARTESIAN_POINT('Origin',(2.2,1.415,12.3105117766515));
#32521=CARTESIAN_POINT('',(2.385,1.415,12.3105117766515));
#32522=CARTESIAN_POINT('Origin',(-4.4,3.185,8.5));
#32523=CARTESIAN_POINT('',(-4.57,3.17,8.5));
#32524=CARTESIAN_POINT('',(-4.585,3.185,8.5));
#32525=CARTESIAN_POINT('',(-4.23,3.17,8.5));
#32526=CARTESIAN_POINT('Origin',(-4.4,3.17,8.5));
#32527=CARTESIAN_POINT('Origin',(-4.4,3.17,8.5));
#32528=CARTESIAN_POINT('Origin',(-4.4,2.275,8.5));
#32529=CARTESIAN_POINT('',(-4.23,1.43,8.5));
#32530=CARTESIAN_POINT('Origin',(-4.4,1.43,8.5));
#32531=CARTESIAN_POINT('',(-4.23,2.275,8.5));
#32532=CARTESIAN_POINT('Origin',(-4.4,1.415,8.5));
#32533=CARTESIAN_POINT('',(-4.215,1.415,8.5));
#32534=CARTESIAN_POINT('Origin',(2.2,3.185,4.68948822334847));
#32535=CARTESIAN_POINT('',(2.03,3.17,4.68948822334847));
#32536=CARTESIAN_POINT('',(2.015,3.185,4.68948822334847));
#32537=CARTESIAN_POINT('',(2.37,3.17,4.68948822334847));
#32538=CARTESIAN_POINT('Origin',(2.2,3.17,4.68948822334847));
#32539=CARTESIAN_POINT('Origin',(2.2,3.17,4.68948822334847));
#32540=CARTESIAN_POINT('Origin',(2.2,2.275,4.68948822334847));
#32541=CARTESIAN_POINT('',(2.37,1.43,4.68948822334847));
#32542=CARTESIAN_POINT('Origin',(2.2,1.43,4.68948822334847));
#32543=CARTESIAN_POINT('',(2.37,2.275,4.68948822334847));
#32544=CARTESIAN_POINT('Origin',(2.2,1.415,4.68948822334847));
#32545=CARTESIAN_POINT('',(2.385,1.415,4.68948822334847));
#32546=CARTESIAN_POINT('Origin',(4.63323591024675,1.415,11.175));
#32547=CARTESIAN_POINT('',(5.03823591024675,1.43,11.175));
#32548=CARTESIAN_POINT('',(5.05323591024675,1.415,11.175));
#32549=CARTESIAN_POINT('Origin',(4.63323591024675,1.43,11.175));
#32550=CARTESIAN_POINT('Origin',(4.63323591024675,2.26,11.175));
#32551=CARTESIAN_POINT('',(5.03823591024675,3.17,11.175));
#32552=CARTESIAN_POINT('',(5.03823591024675,2.26,11.175));
#32553=CARTESIAN_POINT('Origin',(4.63323591024675,3.17,11.175));
#32554=CARTESIAN_POINT('Origin',(-4.63323591024675,1.415,11.175));
#32555=CARTESIAN_POINT('',(-4.22823591024675,1.43,11.175));
#32556=CARTESIAN_POINT('',(-4.21323591024675,1.415,11.175));
#32557=CARTESIAN_POINT('Origin',(-4.63323591024675,1.43,11.175));
#32558=CARTESIAN_POINT('Origin',(-4.63323591024675,2.26,11.175));
#32559=CARTESIAN_POINT('',(-4.22823591024675,3.17,11.175));
#32560=CARTESIAN_POINT('',(-4.22823591024675,2.26,11.175));
#32561=CARTESIAN_POINT('Origin',(-4.63323591024675,3.17,11.175));
#32562=CARTESIAN_POINT('Origin',(-9.82779056315751E-16,1.415,3.15));
#32563=CARTESIAN_POINT('',(0.404999999999999,1.43,3.15));
#32564=CARTESIAN_POINT('',(0.419999999999999,1.415,3.15));
#32565=CARTESIAN_POINT('Origin',(-9.82779056315751E-16,1.43,3.15));
#32566=CARTESIAN_POINT('Origin',(-9.82779056315751E-16,2.26,3.15));
#32567=CARTESIAN_POINT('',(0.404999999999999,3.17,3.15));
#32568=CARTESIAN_POINT('',(0.404999999999999,2.26,3.15));
#32569=CARTESIAN_POINT('Origin',(-9.82779056315751E-16,3.17,3.15));
#32570=CARTESIAN_POINT('Origin',(3.5,2.3,16.1893933982822));
#32571=CARTESIAN_POINT('',(3.015,2.3,16.2));
#32572=CARTESIAN_POINT('Origin',(3.5,2.3,16.2));
#32573=CARTESIAN_POINT('',(3.0662132034356,2.3,16.1787867965644));
#32574=CARTESIAN_POINT('',(3.0406066017178,2.3,16.1893933982822));
#32575=CARTESIAN_POINT('Origin',(3.5,2.3,16.1787867965644));
#32576=CARTESIAN_POINT('Origin',(3.5,2.3,16.2));
#32577=CARTESIAN_POINT('',(3.9262132034356,2.3,16.1712132034356));
#32578=CARTESIAN_POINT('',(3.0737867965644,2.3,16.1712132034356));
#32579=CARTESIAN_POINT('Origin',(3.5,2.3,16.1712132034356));
#32580=CARTESIAN_POINT('Origin',(3.5,2.3,16.1712132034356));
#32581=CARTESIAN_POINT('',(3.045,2.3,16.2));
#32582=CARTESIAN_POINT('Origin',(-6.2,1.4,16.2));
#32583=CARTESIAN_POINT('',(5.6,1.4,16.2));
#32584=CARTESIAN_POINT('Origin',(3.5,2.3,16.1456066017178));
#32585=CARTESIAN_POINT('',(3.905,2.3,16.12));
#32586=CARTESIAN_POINT('',(3.095,2.3,16.12));
#32587=CARTESIAN_POINT('Origin',(3.5,2.3,16.12));
#32588=CARTESIAN_POINT('Origin',(3.5,2.3,16.12));
#32589=CARTESIAN_POINT('',(3.9156066017178,2.3,16.1456066017178));
#32590=CARTESIAN_POINT('Origin',(3.5,2.3,15.675));
#32591=CARTESIAN_POINT('',(3.095,2.3,15.2));
#32592=CARTESIAN_POINT('Origin',(3.5,2.3,15.2));
#32593=CARTESIAN_POINT('',(3.095,2.3,15.675));
#32594=CARTESIAN_POINT('Origin',(3.5,2.3,15.0783257246469));
#32595=CARTESIAN_POINT('',(3.5,2.3,14.9566514492938));
#32596=CARTESIAN_POINT('',(3.2975,2.3,15.0783257246469));
#32597=CARTESIAN_POINT('Origin',(4.5,2.3,2.27660972892601));
#32598=CARTESIAN_POINT('',(4.5,2.3,2.35321945785203));
#32599=CARTESIAN_POINT('',(4.755,2.3,2.2));
#32600=CARTESIAN_POINT('',(4.6275,2.3,2.27660972892601));
#32601=CARTESIAN_POINT('Origin',(4.5,2.3,2.2));
#32602=CARTESIAN_POINT('Origin',(4.5,2.3,1.725));
#32603=CARTESIAN_POINT('',(4.755,2.3,1.25));
#32604=CARTESIAN_POINT('',(4.755,2.3,1.725));
#32605=CARTESIAN_POINT('Origin',(4.5,2.3,1.25));
#32606=CARTESIAN_POINT('Origin',(4.5,2.3,1.2));
#32607=CARTESIAN_POINT('',(4.805,2.3,1.2));
#32608=CARTESIAN_POINT('Origin',(0.,2.3,2.27660972892601));
#32609=CARTESIAN_POINT('',(0.,2.3,2.35321945785203));
#32610=CARTESIAN_POINT('',(0.255,2.3,2.2));
#32611=CARTESIAN_POINT('',(0.1275,2.3,2.27660972892601));
#32612=CARTESIAN_POINT('Origin',(0.,2.3,2.2));
#32613=CARTESIAN_POINT('Origin',(0.,2.3,1.725));
#32614=CARTESIAN_POINT('',(0.255,2.3,1.25));
#32615=CARTESIAN_POINT('',(0.255,2.3,1.725));
#32616=CARTESIAN_POINT('Origin',(0.,2.3,1.25));
#32617=CARTESIAN_POINT('Origin',(0.,2.3,1.2));
#32618=CARTESIAN_POINT('',(0.305,2.3,1.2));
#32619=CARTESIAN_POINT('Origin',(-4.5,2.3,2.27660972892601));
#32620=CARTESIAN_POINT('',(-4.5,2.3,2.35321945785203));
#32621=CARTESIAN_POINT('',(-4.245,2.3,2.2));
#32622=CARTESIAN_POINT('',(-4.3725,2.3,2.27660972892601));
#32623=CARTESIAN_POINT('Origin',(-4.5,2.3,2.2));
#32624=CARTESIAN_POINT('Origin',(-4.5,2.3,1.725));
#32625=CARTESIAN_POINT('',(-4.245,2.3,1.25));
#32626=CARTESIAN_POINT('',(-4.245,2.3,1.725));
#32627=CARTESIAN_POINT('Origin',(-4.5,2.3,1.25));
#32628=CARTESIAN_POINT('Origin',(-4.5,2.3,1.2));
#32629=CARTESIAN_POINT('',(-4.195,2.3,1.2));
#32630=CARTESIAN_POINT('Origin',(-9.82779056315751E-16,3.21,3.15));
#32631=CARTESIAN_POINT('',(0.429999999999999,3.21,3.15));
#32632=CARTESIAN_POINT('Origin',(-4.63323591024675,3.21,11.175));
#32633=CARTESIAN_POINT('',(-4.20323591024675,3.21,11.175));
#32634=CARTESIAN_POINT('Origin',(4.63323591024675,3.21,11.175));
#32635=CARTESIAN_POINT('',(5.06323591024675,3.21,11.175));
#32636=CARTESIAN_POINT('Origin',(-2.2,2.45343330202536,4.68948822334847));
#32637=CARTESIAN_POINT('',(-2.2,2.40686660405073,4.68948822334847));
#32638=CARTESIAN_POINT('',(-2.045,2.5,4.68948822334847));
#32639=CARTESIAN_POINT('',(-2.1225,2.45343330202536,4.68948822334847));
#32640=CARTESIAN_POINT('Origin',(-2.2,2.5,4.68948822334847));
#32641=CARTESIAN_POINT('Origin',(-2.2,2.825,4.68948822334847));
#32642=CARTESIAN_POINT('',(-2.045,3.15,4.68948822334847));
#32643=CARTESIAN_POINT('',(-2.045,2.825,4.68948822334847));
#32644=CARTESIAN_POINT('Origin',(-2.2,3.15,4.68948822334847));
#32645=CARTESIAN_POINT('Origin',(-2.2,3.2,4.68948822334847));
#32646=CARTESIAN_POINT('',(-1.995,3.2,4.68948822334847));
#32647=CARTESIAN_POINT('Origin',(-2.2,2.45343330202536,12.3105117766515));
#32648=CARTESIAN_POINT('',(-2.2,2.40686660405073,12.3105117766515));
#32649=CARTESIAN_POINT('',(-2.045,2.5,12.3105117766515));
#32650=CARTESIAN_POINT('',(-2.1225,2.45343330202536,12.3105117766515));
#32651=CARTESIAN_POINT('Origin',(-2.2,2.5,12.3105117766515));
#32652=CARTESIAN_POINT('Origin',(-2.2,2.825,12.3105117766515));
#32653=CARTESIAN_POINT('',(-2.045,3.15,12.3105117766515));
#32654=CARTESIAN_POINT('',(-2.045,2.825,12.3105117766515));
#32655=CARTESIAN_POINT('Origin',(-2.2,3.15,12.3105117766515));
#32656=CARTESIAN_POINT('Origin',(-2.2,3.2,12.3105117766515));
#32657=CARTESIAN_POINT('',(-1.995,3.2,12.3105117766515));
#32658=CARTESIAN_POINT('Origin',(4.4,2.45343330202536,8.5));
#32659=CARTESIAN_POINT('',(4.4,2.40686660405073,8.5));
#32660=CARTESIAN_POINT('',(4.555,2.5,8.5));
#32661=CARTESIAN_POINT('',(4.4775,2.45343330202536,8.5));
#32662=CARTESIAN_POINT('Origin',(4.4,2.5,8.5));
#32663=CARTESIAN_POINT('Origin',(4.4,2.825,8.5));
#32664=CARTESIAN_POINT('',(4.555,3.15,8.5));
#32665=CARTESIAN_POINT('',(4.555,2.825,8.5));
#32666=CARTESIAN_POINT('Origin',(4.4,3.15,8.5));
#32667=CARTESIAN_POINT('Origin',(4.4,3.2,8.5));
#32668=CARTESIAN_POINT('',(4.605,3.2,8.5));
#32669=CARTESIAN_POINT('Origin',(-3.1,3.16,16.16));
#32670=CARTESIAN_POINT('Origin',(5.6,1.4,15.6));
#53617=UNCERTAINTY_MEASURE_WITH_UNIT(LENGTH_MEASURE(0.001),#53651,
'DISTANCE_ACCURACY_VALUE',
'Maximum model space distance between geometric entities at asserted c
onnectivities');
#53632=UNCERTAINTY_MEASURE_WITH_UNIT(LENGTH_MEASURE(0.001),#53651,
'DISTANCE_ACCURACY_VALUE',
'Maximum model space distance between geometric entities at asserted c
onnectivities');
#53635=(
GEOMETRIC_REPRESENTATION_CONTEXT(3)
GLOBAL_UNCERTAINTY_ASSIGNED_CONTEXT((#53617))
GLOBAL_UNIT_ASSIGNED_CONTEXT((#53651,#53653,#53654))
REPRESENTATION_CONTEXT('','3D')
);
#53650=(
GEOMETRIC_REPRESENTATION_CONTEXT(3)
GLOBAL_UNCERTAINTY_ASSIGNED_CONTEXT((#53632))
GLOBAL_UNIT_ASSIGNED_CONTEXT((#53651,#53653,#53654))
REPRESENTATION_CONTEXT('','3D')
);
#53651=(
LENGTH_UNIT()
NAMED_UNIT(*)
SI_UNIT(.CENTI.,.METRE.)
);
#53653=(
NAMED_UNIT(*)
PLANE_ANGLE_UNIT()
SI_UNIT($,.RADIAN.)
);
#53654=(
NAMED_UNIT(*)
SI_UNIT($,.STERADIAN.)
SOLID_ANGLE_UNIT()
);
#53657=SHAPE_DEFINITION_REPRESENTATION(#53674,#53725);
#53674=PRODUCT_DEFINITION_SHAPE('',$,#53743);
#53725=SHAPE_REPRESENTATION('',(#23686),#53635);
#53740=PRODUCT_DEFINITION_CONTEXT('part definition',#53793,'design');
#53743=PRODUCT_DEFINITION('2026-10-18-22-44-26-297',
'02_Rear_Mirror_Cell_Plate',#53760,#53740);
#53760=PRODUCT_DEFINITION_FORMATION('',$,#53797);
#53793=APPLICATION_CONTEXT(
'Core Data for Automotive Mechanical Design Process');
#53794=PRODUCT_CONTEXT('part definition',#53793,'mechanical');
#53797=PRODUCT('2026-10-18-22-44-26-297','02_Rear_Mirror_Cell_Plate',$,
(#53794));
#53938=COLOUR_RGB('Light Blue',0.38,0.62,0.78);
#53939=FILL_AREA_STYLE_COLOUR('',#53938);
#53940=FILL_AREA_STYLE('',(#53939));
#53941=SURFACE_STYLE_FILL_AREA(#53940);
#53942=SURFACE_SIDE_STYLE('',(#53941));
#53943=SURFACE_STYLE_USAGE(.BOTH.,#53942);
#53944=PRESENTATION_STYLE_ASSIGNMENT((#53943));
ENDSEC;
END-ISO-10303-21;
